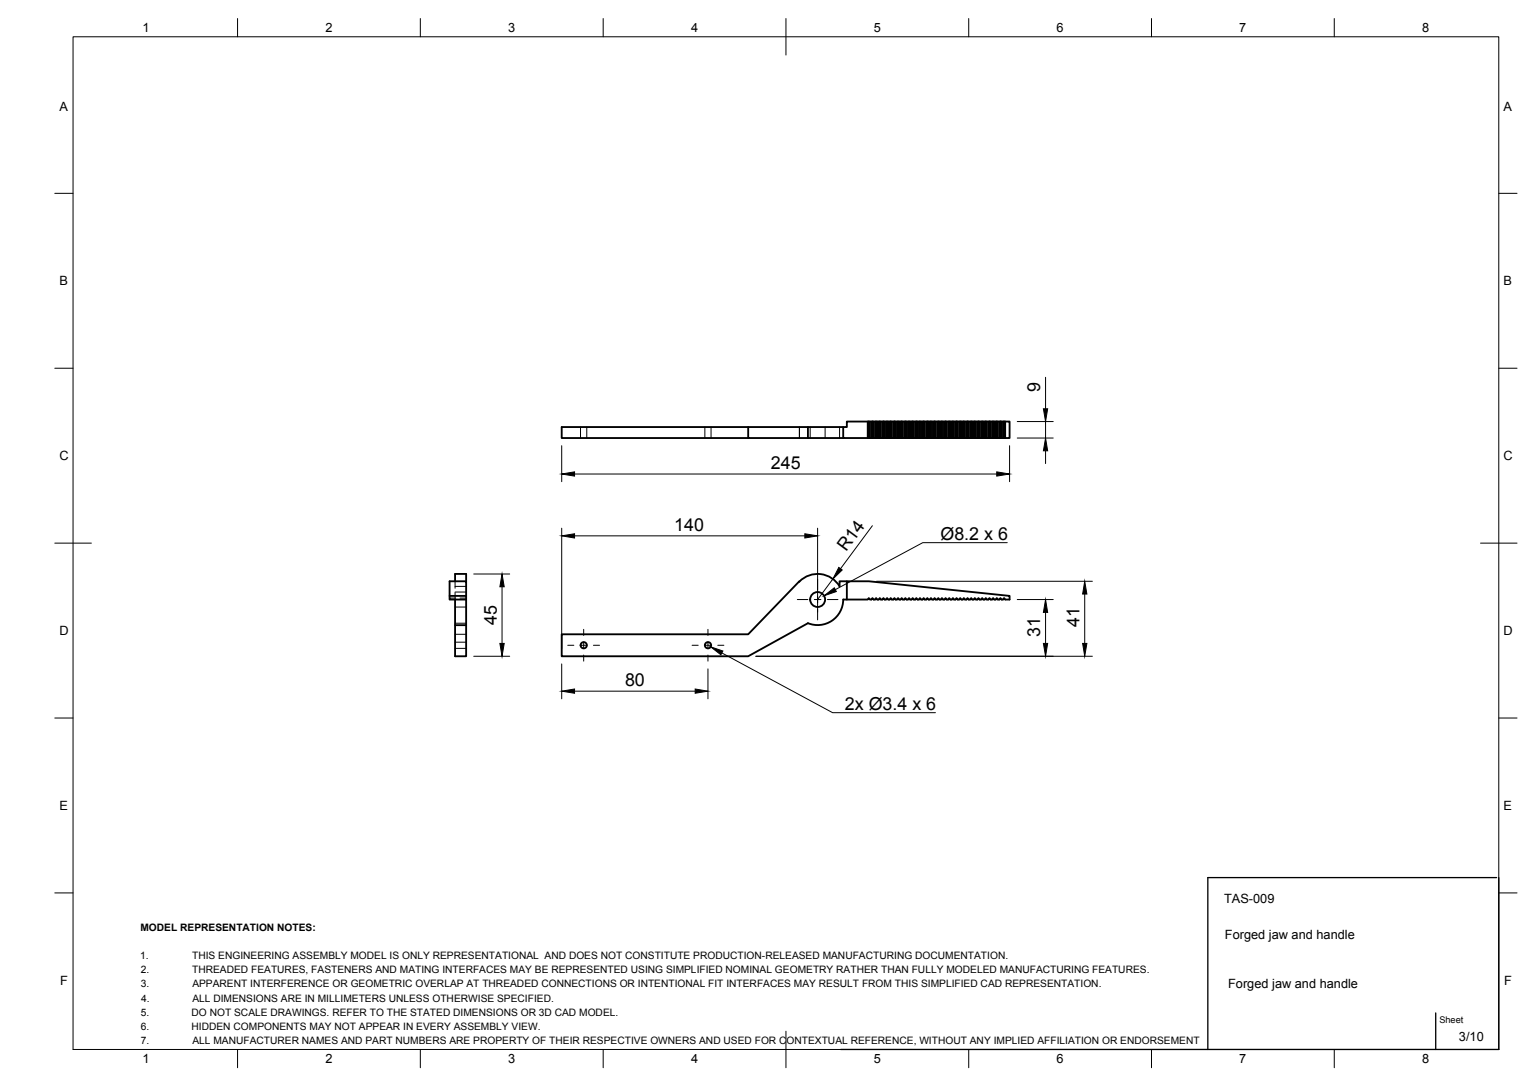
ISO-10303-21;
HEADER;
/* Generated by software containing ST-Developer
 * from STEP Tools, Inc. (www.steptools.com) 
 */

FILE_DESCRIPTION(
/* description */ (''),
/* implementation_level */ '2;1');

FILE_NAME(
/* name */ 'Forged jaw and handle.step',
/* time_stamp */ '2026-11-12T00:53:40-08:00',
/* author */ (''),
/* organization */ (''),
/* preprocessor_version */ 'ST-DEVELOPER v20.2',
/* originating_system */ 'Autodesk Translation Framework v15.17.0.0',
/* authorisation */ '');

FILE_SCHEMA (('AUTOMOTIVE_DESIGN { 1 0 10303 214 3 1 1 }'));
ENDSEC;

DATA;
#10=MECHANICAL_DESIGN_GEOMETRIC_PRESENTATION_REPRESENTATION('',(#572),#22129);
#554=SHAPE_REPRESENTATION_RELATIONSHIP('SRR','None',#22173,#563);
#563=ADVANCED_BREP_SHAPE_REPRESENTATION('',(#581),#22119);
#572=STYLED_ITEM('',(#22232),#581);
#581=MANIFOLD_SOLID_BREP('Body1',#8803);
#590=FACE_BOUND('',#1511,.T.);
#591=FACE_BOUND('',#1512,.T.);
#592=FACE_BOUND('',#1513,.T.);
#593=FACE_BOUND('',#1522,.T.);
#594=FACE_BOUND('',#1523,.T.);
#595=FACE_BOUND('',#1524,.T.);
#651=PLANE('',#8923);
#652=PLANE('',#8924);
#653=PLANE('',#8925);
#654=PLANE('',#8926);
#655=PLANE('',#8927);
#656=PLANE('',#8928);
#657=PLANE('',#8929);
#658=PLANE('',#8930);
#659=PLANE('',#8931);
#660=PLANE('',#8932);
#661=PLANE('',#8933);
#662=PLANE('',#8934);
#663=PLANE('',#8935);
#664=PLANE('',#8936);
#665=PLANE('',#8937);
#666=PLANE('',#8938);
#667=PLANE('',#8939);
#668=PLANE('',#8940);
#669=PLANE('',#8941);
#670=PLANE('',#8942);
#671=PLANE('',#8943);
#672=PLANE('',#8944);
#673=PLANE('',#8945);
#674=PLANE('',#8946);
#675=PLANE('',#8947);
#676=PLANE('',#8948);
#677=PLANE('',#8949);
#678=PLANE('',#8950);
#679=PLANE('',#8951);
#680=PLANE('',#8952);
#681=PLANE('',#8953);
#682=PLANE('',#8954);
#683=PLANE('',#8955);
#684=PLANE('',#8956);
#685=PLANE('',#8957);
#686=PLANE('',#8958);
#687=PLANE('',#8959);
#688=PLANE('',#8960);
#689=PLANE('',#8961);
#690=PLANE('',#8962);
#691=PLANE('',#8963);
#692=PLANE('',#8964);
#693=PLANE('',#8965);
#694=PLANE('',#8966);
#695=PLANE('',#8967);
#696=PLANE('',#8968);
#697=PLANE('',#8969);
#698=PLANE('',#8970);
#699=PLANE('',#8971);
#700=PLANE('',#8972);
#701=PLANE('',#8973);
#702=PLANE('',#8974);
#703=PLANE('',#8975);
#704=PLANE('',#8976);
#705=PLANE('',#8977);
#706=PLANE('',#8978);
#707=PLANE('',#8979);
#708=PLANE('',#8980);
#709=PLANE('',#8981);
#710=PLANE('',#8982);
#711=PLANE('',#8983);
#712=PLANE('',#8984);
#713=PLANE('',#8985);
#714=PLANE('',#8986);
#715=PLANE('',#8987);
#716=PLANE('',#8988);
#717=PLANE('',#8989);
#718=PLANE('',#8990);
#719=PLANE('',#8991);
#720=PLANE('',#8992);
#721=PLANE('',#8993);
#722=PLANE('',#8994);
#723=PLANE('',#8995);
#724=PLANE('',#8996);
#725=PLANE('',#8997);
#726=PLANE('',#8998);
#727=PLANE('',#8999);
#728=PLANE('',#9000);
#729=PLANE('',#9001);
#730=PLANE('',#9002);
#731=PLANE('',#9003);
#732=PLANE('',#9004);
#733=PLANE('',#9005);
#734=PLANE('',#9006);
#735=PLANE('',#9007);
#736=PLANE('',#9008);
#737=PLANE('',#9009);
#738=PLANE('',#9010);
#739=PLANE('',#9011);
#740=PLANE('',#9012);
#741=PLANE('',#9013);
#742=PLANE('',#9014);
#743=PLANE('',#9015);
#744=PLANE('',#9016);
#745=PLANE('',#9017);
#746=PLANE('',#9018);
#747=PLANE('',#9019);
#748=PLANE('',#9020);
#749=PLANE('',#9021);
#750=PLANE('',#9022);
#751=PLANE('',#9023);
#752=PLANE('',#9024);
#753=PLANE('',#9025);
#754=PLANE('',#9026);
#755=PLANE('',#9027);
#756=PLANE('',#9028);
#757=PLANE('',#9029);
#758=PLANE('',#9030);
#759=PLANE('',#9031);
#760=PLANE('',#9032);
#761=PLANE('',#9033);
#762=PLANE('',#9034);
#763=PLANE('',#9035);
#764=PLANE('',#9036);
#765=PLANE('',#9037);
#766=PLANE('',#9038);
#767=PLANE('',#9039);
#768=PLANE('',#9040);
#769=PLANE('',#9041);
#770=PLANE('',#9042);
#771=PLANE('',#9043);
#772=PLANE('',#9044);
#773=PLANE('',#9049);
#774=PLANE('',#9050);
#775=PLANE('',#9051);
#776=PLANE('',#9052);
#777=PLANE('',#9053);
#778=PLANE('',#9054);
#779=PLANE('',#9055);
#903=FACE_OUTER_BOUND('',#1386,.T.);
#904=FACE_OUTER_BOUND('',#1387,.T.);
#905=FACE_OUTER_BOUND('',#1388,.T.);
#906=FACE_OUTER_BOUND('',#1389,.T.);
#907=FACE_OUTER_BOUND('',#1390,.T.);
#908=FACE_OUTER_BOUND('',#1391,.T.);
#909=FACE_OUTER_BOUND('',#1392,.T.);
#910=FACE_OUTER_BOUND('',#1393,.T.);
#911=FACE_OUTER_BOUND('',#1394,.T.);
#912=FACE_OUTER_BOUND('',#1395,.T.);
#913=FACE_OUTER_BOUND('',#1396,.T.);
#914=FACE_OUTER_BOUND('',#1397,.T.);
#915=FACE_OUTER_BOUND('',#1398,.T.);
#916=FACE_OUTER_BOUND('',#1399,.T.);
#917=FACE_OUTER_BOUND('',#1400,.T.);
#918=FACE_OUTER_BOUND('',#1401,.T.);
#919=FACE_OUTER_BOUND('',#1402,.T.);
#920=FACE_OUTER_BOUND('',#1403,.T.);
#921=FACE_OUTER_BOUND('',#1404,.T.);
#922=FACE_OUTER_BOUND('',#1405,.T.);
#923=FACE_OUTER_BOUND('',#1406,.T.);
#924=FACE_OUTER_BOUND('',#1407,.T.);
#925=FACE_OUTER_BOUND('',#1408,.T.);
#926=FACE_OUTER_BOUND('',#1409,.T.);
#927=FACE_OUTER_BOUND('',#1410,.T.);
#928=FACE_OUTER_BOUND('',#1411,.T.);
#929=FACE_OUTER_BOUND('',#1412,.T.);
#930=FACE_OUTER_BOUND('',#1413,.T.);
#931=FACE_OUTER_BOUND('',#1414,.T.);
#932=FACE_OUTER_BOUND('',#1415,.T.);
#933=FACE_OUTER_BOUND('',#1416,.T.);
#934=FACE_OUTER_BOUND('',#1417,.T.);
#935=FACE_OUTER_BOUND('',#1418,.T.);
#936=FACE_OUTER_BOUND('',#1419,.T.);
#937=FACE_OUTER_BOUND('',#1420,.T.);
#938=FACE_OUTER_BOUND('',#1421,.T.);
#939=FACE_OUTER_BOUND('',#1422,.T.);
#940=FACE_OUTER_BOUND('',#1423,.T.);
#941=FACE_OUTER_BOUND('',#1424,.T.);
#942=FACE_OUTER_BOUND('',#1425,.T.);
#943=FACE_OUTER_BOUND('',#1426,.T.);
#944=FACE_OUTER_BOUND('',#1427,.T.);
#945=FACE_OUTER_BOUND('',#1428,.T.);
#946=FACE_OUTER_BOUND('',#1429,.T.);
#947=FACE_OUTER_BOUND('',#1430,.T.);
#948=FACE_OUTER_BOUND('',#1431,.T.);
#949=FACE_OUTER_BOUND('',#1432,.T.);
#950=FACE_OUTER_BOUND('',#1433,.T.);
#951=FACE_OUTER_BOUND('',#1434,.T.);
#952=FACE_OUTER_BOUND('',#1435,.T.);
#953=FACE_OUTER_BOUND('',#1436,.T.);
#954=FACE_OUTER_BOUND('',#1437,.T.);
#955=FACE_OUTER_BOUND('',#1438,.T.);
#956=FACE_OUTER_BOUND('',#1439,.T.);
#957=FACE_OUTER_BOUND('',#1440,.T.);
#958=FACE_OUTER_BOUND('',#1441,.T.);
#959=FACE_OUTER_BOUND('',#1442,.T.);
#960=FACE_OUTER_BOUND('',#1443,.T.);
#961=FACE_OUTER_BOUND('',#1444,.T.);
#962=FACE_OUTER_BOUND('',#1445,.T.);
#963=FACE_OUTER_BOUND('',#1446,.T.);
#964=FACE_OUTER_BOUND('',#1447,.T.);
#965=FACE_OUTER_BOUND('',#1448,.T.);
#966=FACE_OUTER_BOUND('',#1449,.T.);
#967=FACE_OUTER_BOUND('',#1450,.T.);
#968=FACE_OUTER_BOUND('',#1451,.T.);
#969=FACE_OUTER_BOUND('',#1452,.T.);
#970=FACE_OUTER_BOUND('',#1453,.T.);
#971=FACE_OUTER_BOUND('',#1454,.T.);
#972=FACE_OUTER_BOUND('',#1455,.T.);
#973=FACE_OUTER_BOUND('',#1456,.T.);
#974=FACE_OUTER_BOUND('',#1457,.T.);
#975=FACE_OUTER_BOUND('',#1458,.T.);
#976=FACE_OUTER_BOUND('',#1459,.T.);
#977=FACE_OUTER_BOUND('',#1460,.T.);
#978=FACE_OUTER_BOUND('',#1461,.T.);
#979=FACE_OUTER_BOUND('',#1462,.T.);
#980=FACE_OUTER_BOUND('',#1463,.T.);
#981=FACE_OUTER_BOUND('',#1464,.T.);
#982=FACE_OUTER_BOUND('',#1465,.T.);
#983=FACE_OUTER_BOUND('',#1466,.T.);
#984=FACE_OUTER_BOUND('',#1467,.T.);
#985=FACE_OUTER_BOUND('',#1468,.T.);
#986=FACE_OUTER_BOUND('',#1469,.T.);
#987=FACE_OUTER_BOUND('',#1470,.T.);
#988=FACE_OUTER_BOUND('',#1471,.T.);
#989=FACE_OUTER_BOUND('',#1472,.T.);
#990=FACE_OUTER_BOUND('',#1473,.T.);
#991=FACE_OUTER_BOUND('',#1474,.T.);
#992=FACE_OUTER_BOUND('',#1475,.T.);
#993=FACE_OUTER_BOUND('',#1476,.T.);
#994=FACE_OUTER_BOUND('',#1477,.T.);
#995=FACE_OUTER_BOUND('',#1478,.T.);
#996=FACE_OUTER_BOUND('',#1479,.T.);
#997=FACE_OUTER_BOUND('',#1480,.T.);
#998=FACE_OUTER_BOUND('',#1481,.T.);
#999=FACE_OUTER_BOUND('',#1482,.T.);
#1000=FACE_OUTER_BOUND('',#1483,.T.);
#1001=FACE_OUTER_BOUND('',#1484,.T.);
#1002=FACE_OUTER_BOUND('',#1485,.T.);
#1003=FACE_OUTER_BOUND('',#1486,.T.);
#1004=FACE_OUTER_BOUND('',#1487,.T.);
#1005=FACE_OUTER_BOUND('',#1488,.T.);
#1006=FACE_OUTER_BOUND('',#1489,.T.);
#1007=FACE_OUTER_BOUND('',#1490,.T.);
#1008=FACE_OUTER_BOUND('',#1491,.T.);
#1009=FACE_OUTER_BOUND('',#1492,.T.);
#1010=FACE_OUTER_BOUND('',#1493,.T.);
#1011=FACE_OUTER_BOUND('',#1494,.T.);
#1012=FACE_OUTER_BOUND('',#1495,.T.);
#1013=FACE_OUTER_BOUND('',#1496,.T.);
#1014=FACE_OUTER_BOUND('',#1497,.T.);
#1015=FACE_OUTER_BOUND('',#1498,.T.);
#1016=FACE_OUTER_BOUND('',#1499,.T.);
#1017=FACE_OUTER_BOUND('',#1500,.T.);
#1018=FACE_OUTER_BOUND('',#1501,.T.);
#1019=FACE_OUTER_BOUND('',#1502,.T.);
#1020=FACE_OUTER_BOUND('',#1503,.T.);
#1021=FACE_OUTER_BOUND('',#1504,.T.);
#1022=FACE_OUTER_BOUND('',#1505,.T.);
#1023=FACE_OUTER_BOUND('',#1506,.T.);
#1024=FACE_OUTER_BOUND('',#1507,.T.);
#1025=FACE_OUTER_BOUND('',#1508,.T.);
#1026=FACE_OUTER_BOUND('',#1509,.T.);
#1027=FACE_OUTER_BOUND('',#1510,.T.);
#1028=FACE_OUTER_BOUND('',#1514,.T.);
#1029=FACE_OUTER_BOUND('',#1515,.T.);
#1030=FACE_OUTER_BOUND('',#1516,.T.);
#1031=FACE_OUTER_BOUND('',#1517,.T.);
#1032=FACE_OUTER_BOUND('',#1518,.T.);
#1033=FACE_OUTER_BOUND('',#1519,.T.);
#1034=FACE_OUTER_BOUND('',#1520,.T.);
#1035=FACE_OUTER_BOUND('',#1521,.T.);
#1036=FACE_OUTER_BOUND('',#1525,.T.);
#1386=EDGE_LOOP('',(#5646,#5647,#5648,#5649));
#1387=EDGE_LOOP('',(#5650,#5651,#5652,#5653));
#1388=EDGE_LOOP('',(#5654,#5655,#5656,#5657));
#1389=EDGE_LOOP('',(#5658,#5659,#5660,#5661));
#1390=EDGE_LOOP('',(#5662,#5663,#5664,#5665));
#1391=EDGE_LOOP('',(#5666,#5667,#5668,#5669));
#1392=EDGE_LOOP('',(#5670,#5671,#5672,#5673));
#1393=EDGE_LOOP('',(#5674,#5675,#5676,#5677));
#1394=EDGE_LOOP('',(#5678,#5679,#5680,#5681));
#1395=EDGE_LOOP('',(#5682,#5683,#5684,#5685));
#1396=EDGE_LOOP('',(#5686,#5687,#5688,#5689));
#1397=EDGE_LOOP('',(#5690,#5691,#5692,#5693));
#1398=EDGE_LOOP('',(#5694,#5695,#5696,#5697));
#1399=EDGE_LOOP('',(#5698,#5699,#5700,#5701));
#1400=EDGE_LOOP('',(#5702,#5703,#5704,#5705));
#1401=EDGE_LOOP('',(#5706,#5707,#5708,#5709));
#1402=EDGE_LOOP('',(#5710,#5711,#5712,#5713));
#1403=EDGE_LOOP('',(#5714,#5715,#5716,#5717));
#1404=EDGE_LOOP('',(#5718,#5719,#5720,#5721));
#1405=EDGE_LOOP('',(#5722,#5723,#5724,#5725));
#1406=EDGE_LOOP('',(#5726,#5727,#5728,#5729));
#1407=EDGE_LOOP('',(#5730,#5731,#5732,#5733));
#1408=EDGE_LOOP('',(#5734,#5735,#5736,#5737));
#1409=EDGE_LOOP('',(#5738,#5739,#5740,#5741));
#1410=EDGE_LOOP('',(#5742,#5743,#5744,#5745));
#1411=EDGE_LOOP('',(#5746,#5747,#5748,#5749));
#1412=EDGE_LOOP('',(#5750,#5751,#5752,#5753));
#1413=EDGE_LOOP('',(#5754,#5755,#5756,#5757));
#1414=EDGE_LOOP('',(#5758,#5759,#5760,#5761));
#1415=EDGE_LOOP('',(#5762,#5763,#5764,#5765));
#1416=EDGE_LOOP('',(#5766,#5767,#5768,#5769));
#1417=EDGE_LOOP('',(#5770,#5771,#5772,#5773));
#1418=EDGE_LOOP('',(#5774,#5775,#5776,#5777));
#1419=EDGE_LOOP('',(#5778,#5779,#5780,#5781));
#1420=EDGE_LOOP('',(#5782,#5783,#5784,#5785));
#1421=EDGE_LOOP('',(#5786,#5787,#5788,#5789));
#1422=EDGE_LOOP('',(#5790,#5791,#5792,#5793));
#1423=EDGE_LOOP('',(#5794,#5795,#5796,#5797));
#1424=EDGE_LOOP('',(#5798,#5799,#5800,#5801));
#1425=EDGE_LOOP('',(#5802,#5803,#5804,#5805));
#1426=EDGE_LOOP('',(#5806,#5807,#5808,#5809));
#1427=EDGE_LOOP('',(#5810,#5811,#5812,#5813));
#1428=EDGE_LOOP('',(#5814,#5815,#5816,#5817));
#1429=EDGE_LOOP('',(#5818,#5819,#5820,#5821));
#1430=EDGE_LOOP('',(#5822,#5823,#5824,#5825));
#1431=EDGE_LOOP('',(#5826,#5827,#5828,#5829));
#1432=EDGE_LOOP('',(#5830,#5831,#5832,#5833));
#1433=EDGE_LOOP('',(#5834,#5835,#5836,#5837));
#1434=EDGE_LOOP('',(#5838,#5839,#5840,#5841));
#1435=EDGE_LOOP('',(#5842,#5843,#5844,#5845));
#1436=EDGE_LOOP('',(#5846,#5847,#5848,#5849));
#1437=EDGE_LOOP('',(#5850,#5851,#5852,#5853));
#1438=EDGE_LOOP('',(#5854,#5855,#5856,#5857));
#1439=EDGE_LOOP('',(#5858,#5859,#5860,#5861));
#1440=EDGE_LOOP('',(#5862,#5863,#5864,#5865));
#1441=EDGE_LOOP('',(#5866,#5867,#5868,#5869));
#1442=EDGE_LOOP('',(#5870,#5871,#5872,#5873));
#1443=EDGE_LOOP('',(#5874,#5875,#5876,#5877));
#1444=EDGE_LOOP('',(#5878,#5879,#5880,#5881));
#1445=EDGE_LOOP('',(#5882,#5883,#5884,#5885));
#1446=EDGE_LOOP('',(#5886,#5887,#5888,#5889));
#1447=EDGE_LOOP('',(#5890,#5891,#5892,#5893));
#1448=EDGE_LOOP('',(#5894,#5895,#5896,#5897));
#1449=EDGE_LOOP('',(#5898,#5899,#5900,#5901));
#1450=EDGE_LOOP('',(#5902,#5903,#5904,#5905));
#1451=EDGE_LOOP('',(#5906,#5907,#5908,#5909));
#1452=EDGE_LOOP('',(#5910,#5911,#5912,#5913));
#1453=EDGE_LOOP('',(#5914,#5915,#5916,#5917));
#1454=EDGE_LOOP('',(#5918,#5919,#5920,#5921));
#1455=EDGE_LOOP('',(#5922,#5923,#5924,#5925));
#1456=EDGE_LOOP('',(#5926,#5927,#5928,#5929));
#1457=EDGE_LOOP('',(#5930,#5931,#5932,#5933));
#1458=EDGE_LOOP('',(#5934,#5935,#5936,#5937));
#1459=EDGE_LOOP('',(#5938,#5939,#5940,#5941));
#1460=EDGE_LOOP('',(#5942,#5943,#5944,#5945));
#1461=EDGE_LOOP('',(#5946,#5947,#5948,#5949));
#1462=EDGE_LOOP('',(#5950,#5951,#5952,#5953));
#1463=EDGE_LOOP('',(#5954,#5955,#5956,#5957));
#1464=EDGE_LOOP('',(#5958,#5959,#5960,#5961));
#1465=EDGE_LOOP('',(#5962,#5963,#5964,#5965,#5966,#5967));
#1466=EDGE_LOOP('',(#5968,#5969,#5970,#5971));
#1467=EDGE_LOOP('',(#5972,#5973,#5974,#5975));
#1468=EDGE_LOOP('',(#5976,#5977,#5978,#5979));
#1469=EDGE_LOOP('',(#5980,#5981,#5982,#5983));
#1470=EDGE_LOOP('',(#5984,#5985,#5986,#5987));
#1471=EDGE_LOOP('',(#5988,#5989,#5990,#5991));
#1472=EDGE_LOOP('',(#5992,#5993,#5994,#5995));
#1473=EDGE_LOOP('',(#5996,#5997,#5998,#5999));
#1474=EDGE_LOOP('',(#6000,#6001,#6002,#6003));
#1475=EDGE_LOOP('',(#6004,#6005,#6006,#6007));
#1476=EDGE_LOOP('',(#6008,#6009,#6010,#6011));
#1477=EDGE_LOOP('',(#6012,#6013,#6014,#6015));
#1478=EDGE_LOOP('',(#6016,#6017,#6018,#6019));
#1479=EDGE_LOOP('',(#6020,#6021,#6022,#6023));
#1480=EDGE_LOOP('',(#6024,#6025,#6026,#6027));
#1481=EDGE_LOOP('',(#6028,#6029,#6030,#6031));
#1482=EDGE_LOOP('',(#6032,#6033,#6034,#6035));
#1483=EDGE_LOOP('',(#6036,#6037,#6038,#6039));
#1484=EDGE_LOOP('',(#6040,#6041,#6042,#6043));
#1485=EDGE_LOOP('',(#6044,#6045,#6046,#6047));
#1486=EDGE_LOOP('',(#6048,#6049,#6050,#6051));
#1487=EDGE_LOOP('',(#6052,#6053,#6054,#6055));
#1488=EDGE_LOOP('',(#6056,#6057,#6058,#6059));
#1489=EDGE_LOOP('',(#6060,#6061,#6062,#6063));
#1490=EDGE_LOOP('',(#6064,#6065,#6066,#6067));
#1491=EDGE_LOOP('',(#6068,#6069,#6070,#6071));
#1492=EDGE_LOOP('',(#6072,#6073,#6074,#6075));
#1493=EDGE_LOOP('',(#6076,#6077,#6078,#6079));
#1494=EDGE_LOOP('',(#6080,#6081,#6082,#6083));
#1495=EDGE_LOOP('',(#6084,#6085,#6086,#6087));
#1496=EDGE_LOOP('',(#6088,#6089,#6090,#6091));
#1497=EDGE_LOOP('',(#6092,#6093,#6094,#6095));
#1498=EDGE_LOOP('',(#6096,#6097,#6098,#6099));
#1499=EDGE_LOOP('',(#6100,#6101,#6102,#6103));
#1500=EDGE_LOOP('',(#6104,#6105,#6106,#6107));
#1501=EDGE_LOOP('',(#6108,#6109,#6110,#6111));
#1502=EDGE_LOOP('',(#6112,#6113,#6114,#6115));
#1503=EDGE_LOOP('',(#6116,#6117,#6118,#6119));
#1504=EDGE_LOOP('',(#6120,#6121,#6122,#6123,#6124,#6125,#6126,#6127,#6128,
#6129,#6130,#6131,#6132,#6133,#6134,#6135,#6136,#6137,#6138,#6139,#6140,
#6141,#6142,#6143,#6144,#6145,#6146,#6147,#6148,#6149,#6150,#6151,#6152,
#6153,#6154,#6155,#6156,#6157,#6158,#6159,#6160,#6161,#6162,#6163,#6164,
#6165,#6166,#6167,#6168,#6169,#6170,#6171,#6172,#6173,#6174,#6175,#6176,
#6177,#6178,#6179,#6180,#6181,#6182,#6183,#6184,#6185,#6186,#6187,#6188,
#6189,#6190,#6191,#6192,#6193,#6194,#6195,#6196,#6197,#6198,#6199,#6200,
#6201,#6202,#6203,#6204,#6205,#6206,#6207,#6208,#6209,#6210,#6211,#6212,
#6213,#6214,#6215,#6216,#6217,#6218,#6219,#6220,#6221,#6222,#6223,#6224,
#6225,#6226,#6227,#6228,#6229,#6230,#6231,#6232,#6233,#6234,#6235,#6236,
#6237,#6238));
#1505=EDGE_LOOP('',(#6239,#6240,#6241,#6242));
#1506=EDGE_LOOP('',(#6243,#6244,#6245,#6246));
#1507=EDGE_LOOP('',(#6247,#6248,#6249,#6250));
#1508=EDGE_LOOP('',(#6251,#6252,#6253,#6254));
#1509=EDGE_LOOP('',(#6255,#6256,#6257,#6258,#6259,#6260));
#1510=EDGE_LOOP('',(#6261,#6262,#6263,#6264,#6265,#6266,#6267,#6268,#6269,
#6270,#6271,#6272));
#1511=EDGE_LOOP('',(#6273));
#1512=EDGE_LOOP('',(#6274));
#1513=EDGE_LOOP('',(#6275));
#1514=EDGE_LOOP('',(#6276,#6277,#6278,#6279));
#1515=EDGE_LOOP('',(#6280,#6281,#6282,#6283));
#1516=EDGE_LOOP('',(#6284,#6285,#6286,#6287));
#1517=EDGE_LOOP('',(#6288,#6289,#6290,#6291));
#1518=EDGE_LOOP('',(#6292,#6293,#6294,#6295));
#1519=EDGE_LOOP('',(#6296,#6297,#6298,#6299));
#1520=EDGE_LOOP('',(#6300,#6301,#6302,#6303));
#1521=EDGE_LOOP('',(#6304,#6305,#6306,#6307,#6308,#6309,#6310,#6311,#6312,
#6313,#6314,#6315,#6316,#6317,#6318,#6319,#6320,#6321,#6322,#6323,#6324,
#6325,#6326,#6327,#6328,#6329,#6330,#6331,#6332,#6333,#6334,#6335,#6336,
#6337,#6338,#6339,#6340,#6341,#6342,#6343,#6344,#6345,#6346,#6347,#6348,
#6349,#6350,#6351,#6352,#6353,#6354,#6355,#6356,#6357,#6358,#6359,#6360,
#6361,#6362,#6363,#6364,#6365,#6366,#6367,#6368,#6369,#6370,#6371,#6372,
#6373,#6374,#6375,#6376,#6377,#6378,#6379,#6380,#6381,#6382,#6383,#6384,
#6385,#6386,#6387,#6388,#6389,#6390,#6391,#6392,#6393,#6394,#6395,#6396,
#6397,#6398,#6399,#6400,#6401,#6402,#6403,#6404,#6405,#6406,#6407,#6408,
#6409,#6410,#6411,#6412,#6413,#6414,#6415,#6416,#6417,#6418,#6419,#6420,
#6421,#6422,#6423,#6424,#6425,#6426,#6427,#6428,#6429,#6430));
#1522=EDGE_LOOP('',(#6431));
#1523=EDGE_LOOP('',(#6432));
#1524=EDGE_LOOP('',(#6433));
#1525=EDGE_LOOP('',(#6434,#6435,#6436,#6437));
#1930=LINE('',#11412,#2660);
#1931=LINE('',#11418,#2661);
#1932=LINE('',#11424,#2662);
#1933=LINE('',#11429,#2663);
#1934=LINE('',#11431,#2664);
#1935=LINE('',#11433,#2665);
#1936=LINE('',#11434,#2666);
#1937=LINE('',#11438,#2667);
#1938=LINE('',#11439,#2668);
#1939=LINE('',#11440,#2669);
#1940=LINE('',#11444,#2670);
#1941=LINE('',#11446,#2671);
#1942=LINE('',#11448,#2672);
#1943=LINE('',#11449,#2673);
#1944=LINE('',#11453,#2674);
#1945=LINE('',#11454,#2675);
#1946=LINE('',#11455,#2676);
#1947=LINE('',#11459,#2677);
#1948=LINE('',#11461,#2678);
#1949=LINE('',#11463,#2679);
#1950=LINE('',#11464,#2680);
#1951=LINE('',#11468,#2681);
#1952=LINE('',#11469,#2682);
#1953=LINE('',#11470,#2683);
#1954=LINE('',#11474,#2684);
#1955=LINE('',#11476,#2685);
#1956=LINE('',#11478,#2686);
#1957=LINE('',#11479,#2687);
#1958=LINE('',#11483,#2688);
#1959=LINE('',#11484,#2689);
#1960=LINE('',#11485,#2690);
#1961=LINE('',#11489,#2691);
#1962=LINE('',#11491,#2692);
#1963=LINE('',#11493,#2693);
#1964=LINE('',#11494,#2694);
#1965=LINE('',#11498,#2695);
#1966=LINE('',#11499,#2696);
#1967=LINE('',#11500,#2697);
#1968=LINE('',#11504,#2698);
#1969=LINE('',#11506,#2699);
#1970=LINE('',#11508,#2700);
#1971=LINE('',#11509,#2701);
#1972=LINE('',#11513,#2702);
#1973=LINE('',#11514,#2703);
#1974=LINE('',#11515,#2704);
#1975=LINE('',#11519,#2705);
#1976=LINE('',#11521,#2706);
#1977=LINE('',#11523,#2707);
#1978=LINE('',#11524,#2708);
#1979=LINE('',#11528,#2709);
#1980=LINE('',#11529,#2710);
#1981=LINE('',#11530,#2711);
#1982=LINE('',#11534,#2712);
#1983=LINE('',#11536,#2713);
#1984=LINE('',#11538,#2714);
#1985=LINE('',#11539,#2715);
#1986=LINE('',#11543,#2716);
#1987=LINE('',#11544,#2717);
#1988=LINE('',#11545,#2718);
#1989=LINE('',#11549,#2719);
#1990=LINE('',#11551,#2720);
#1991=LINE('',#11553,#2721);
#1992=LINE('',#11554,#2722);
#1993=LINE('',#11558,#2723);
#1994=LINE('',#11559,#2724);
#1995=LINE('',#11560,#2725);
#1996=LINE('',#11564,#2726);
#1997=LINE('',#11566,#2727);
#1998=LINE('',#11568,#2728);
#1999=LINE('',#11569,#2729);
#2000=LINE('',#11573,#2730);
#2001=LINE('',#11574,#2731);
#2002=LINE('',#11575,#2732);
#2003=LINE('',#11579,#2733);
#2004=LINE('',#11581,#2734);
#2005=LINE('',#11583,#2735);
#2006=LINE('',#11584,#2736);
#2007=LINE('',#11588,#2737);
#2008=LINE('',#11589,#2738);
#2009=LINE('',#11590,#2739);
#2010=LINE('',#11594,#2740);
#2011=LINE('',#11596,#2741);
#2012=LINE('',#11598,#2742);
#2013=LINE('',#11599,#2743);
#2014=LINE('',#11603,#2744);
#2015=LINE('',#11604,#2745);
#2016=LINE('',#11605,#2746);
#2017=LINE('',#11609,#2747);
#2018=LINE('',#11611,#2748);
#2019=LINE('',#11613,#2749);
#2020=LINE('',#11614,#2750);
#2021=LINE('',#11618,#2751);
#2022=LINE('',#11619,#2752);
#2023=LINE('',#11620,#2753);
#2024=LINE('',#11624,#2754);
#2025=LINE('',#11626,#2755);
#2026=LINE('',#11628,#2756);
#2027=LINE('',#11629,#2757);
#2028=LINE('',#11633,#2758);
#2029=LINE('',#11634,#2759);
#2030=LINE('',#11635,#2760);
#2031=LINE('',#11639,#2761);
#2032=LINE('',#11641,#2762);
#2033=LINE('',#11643,#2763);
#2034=LINE('',#11644,#2764);
#2035=LINE('',#11648,#2765);
#2036=LINE('',#11649,#2766);
#2037=LINE('',#11650,#2767);
#2038=LINE('',#11654,#2768);
#2039=LINE('',#11656,#2769);
#2040=LINE('',#11658,#2770);
#2041=LINE('',#11659,#2771);
#2042=LINE('',#11663,#2772);
#2043=LINE('',#11664,#2773);
#2044=LINE('',#11665,#2774);
#2045=LINE('',#11669,#2775);
#2046=LINE('',#11671,#2776);
#2047=LINE('',#11673,#2777);
#2048=LINE('',#11674,#2778);
#2049=LINE('',#11678,#2779);
#2050=LINE('',#11679,#2780);
#2051=LINE('',#11680,#2781);
#2052=LINE('',#11684,#2782);
#2053=LINE('',#11686,#2783);
#2054=LINE('',#11688,#2784);
#2055=LINE('',#11689,#2785);
#2056=LINE('',#11693,#2786);
#2057=LINE('',#11694,#2787);
#2058=LINE('',#11695,#2788);
#2059=LINE('',#11699,#2789);
#2060=LINE('',#11701,#2790);
#2061=LINE('',#11703,#2791);
#2062=LINE('',#11704,#2792);
#2063=LINE('',#11708,#2793);
#2064=LINE('',#11709,#2794);
#2065=LINE('',#11710,#2795);
#2066=LINE('',#11714,#2796);
#2067=LINE('',#11716,#2797);
#2068=LINE('',#11718,#2798);
#2069=LINE('',#11719,#2799);
#2070=LINE('',#11723,#2800);
#2071=LINE('',#11724,#2801);
#2072=LINE('',#11725,#2802);
#2073=LINE('',#11729,#2803);
#2074=LINE('',#11731,#2804);
#2075=LINE('',#11733,#2805);
#2076=LINE('',#11734,#2806);
#2077=LINE('',#11738,#2807);
#2078=LINE('',#11739,#2808);
#2079=LINE('',#11740,#2809);
#2080=LINE('',#11744,#2810);
#2081=LINE('',#11746,#2811);
#2082=LINE('',#11748,#2812);
#2083=LINE('',#11749,#2813);
#2084=LINE('',#11753,#2814);
#2085=LINE('',#11754,#2815);
#2086=LINE('',#11755,#2816);
#2087=LINE('',#11759,#2817);
#2088=LINE('',#11761,#2818);
#2089=LINE('',#11763,#2819);
#2090=LINE('',#11764,#2820);
#2091=LINE('',#11768,#2821);
#2092=LINE('',#11769,#2822);
#2093=LINE('',#11770,#2823);
#2094=LINE('',#11774,#2824);
#2095=LINE('',#11776,#2825);
#2096=LINE('',#11778,#2826);
#2097=LINE('',#11779,#2827);
#2098=LINE('',#11783,#2828);
#2099=LINE('',#11784,#2829);
#2100=LINE('',#11785,#2830);
#2101=LINE('',#11789,#2831);
#2102=LINE('',#11791,#2832);
#2103=LINE('',#11793,#2833);
#2104=LINE('',#11794,#2834);
#2105=LINE('',#11798,#2835);
#2106=LINE('',#11799,#2836);
#2107=LINE('',#11800,#2837);
#2108=LINE('',#11804,#2838);
#2109=LINE('',#11806,#2839);
#2110=LINE('',#11808,#2840);
#2111=LINE('',#11809,#2841);
#2112=LINE('',#11813,#2842);
#2113=LINE('',#11814,#2843);
#2114=LINE('',#11815,#2844);
#2115=LINE('',#11819,#2845);
#2116=LINE('',#11821,#2846);
#2117=LINE('',#11823,#2847);
#2118=LINE('',#11824,#2848);
#2119=LINE('',#11828,#2849);
#2120=LINE('',#11829,#2850);
#2121=LINE('',#11830,#2851);
#2122=LINE('',#11834,#2852);
#2123=LINE('',#11836,#2853);
#2124=LINE('',#11838,#2854);
#2125=LINE('',#11839,#2855);
#2126=LINE('',#11843,#2856);
#2127=LINE('',#11844,#2857);
#2128=LINE('',#11845,#2858);
#2129=LINE('',#11849,#2859);
#2130=LINE('',#11851,#2860);
#2131=LINE('',#11853,#2861);
#2132=LINE('',#11854,#2862);
#2133=LINE('',#11858,#2863);
#2134=LINE('',#11859,#2864);
#2135=LINE('',#11860,#2865);
#2136=LINE('',#11864,#2866);
#2137=LINE('',#11866,#2867);
#2138=LINE('',#11868,#2868);
#2139=LINE('',#11869,#2869);
#2140=LINE('',#11873,#2870);
#2141=LINE('',#11874,#2871);
#2142=LINE('',#11875,#2872);
#2143=LINE('',#11879,#2873);
#2144=LINE('',#11881,#2874);
#2145=LINE('',#11883,#2875);
#2146=LINE('',#11884,#2876);
#2147=LINE('',#11888,#2877);
#2148=LINE('',#11889,#2878);
#2149=LINE('',#11890,#2879);
#2150=LINE('',#11894,#2880);
#2151=LINE('',#11896,#2881);
#2152=LINE('',#11898,#2882);
#2153=LINE('',#11899,#2883);
#2154=LINE('',#11903,#2884);
#2155=LINE('',#11904,#2885);
#2156=LINE('',#11905,#2886);
#2157=LINE('',#11909,#2887);
#2158=LINE('',#11911,#2888);
#2159=LINE('',#11913,#2889);
#2160=LINE('',#11914,#2890);
#2161=LINE('',#11918,#2891);
#2162=LINE('',#11919,#2892);
#2163=LINE('',#11920,#2893);
#2164=LINE('',#11924,#2894);
#2165=LINE('',#11926,#2895);
#2166=LINE('',#11928,#2896);
#2167=LINE('',#11929,#2897);
#2168=LINE('',#11933,#2898);
#2169=LINE('',#11934,#2899);
#2170=LINE('',#11935,#2900);
#2171=LINE('',#11939,#2901);
#2172=LINE('',#11941,#2902);
#2173=LINE('',#11943,#2903);
#2174=LINE('',#11944,#2904);
#2175=LINE('',#11948,#2905);
#2176=LINE('',#11949,#2906);
#2177=LINE('',#11950,#2907);
#2178=LINE('',#11954,#2908);
#2179=LINE('',#11956,#2909);
#2180=LINE('',#11958,#2910);
#2181=LINE('',#11959,#2911);
#2182=LINE('',#11963,#2912);
#2183=LINE('',#11964,#2913);
#2184=LINE('',#11965,#2914);
#2185=LINE('',#11969,#2915);
#2186=LINE('',#11971,#2916);
#2187=LINE('',#11973,#2917);
#2188=LINE('',#11974,#2918);
#2189=LINE('',#11978,#2919);
#2190=LINE('',#11979,#2920);
#2191=LINE('',#11980,#2921);
#2192=LINE('',#11984,#2922);
#2193=LINE('',#11986,#2923);
#2194=LINE('',#11988,#2924);
#2195=LINE('',#11989,#2925);
#2196=LINE('',#11993,#2926);
#2197=LINE('',#11994,#2927);
#2198=LINE('',#11995,#2928);
#2199=LINE('',#11998,#2929);
#2200=LINE('',#12000,#2930);
#2201=LINE('',#12002,#2931);
#2202=LINE('',#12004,#2932);
#2203=LINE('',#12005,#2933);
#2204=LINE('',#12007,#2934);
#2205=LINE('',#12008,#2935);
#2206=LINE('',#12010,#2936);
#2207=LINE('',#12011,#2937);
#2208=LINE('',#12013,#2938);
#2209=LINE('',#12014,#2939);
#2210=LINE('',#12016,#2940);
#2211=LINE('',#12017,#2941);
#2212=LINE('',#12019,#2942);
#2213=LINE('',#12020,#2943);
#2214=LINE('',#12022,#2944);
#2215=LINE('',#12023,#2945);
#2216=LINE('',#12025,#2946);
#2217=LINE('',#12026,#2947);
#2218=LINE('',#12028,#2948);
#2219=LINE('',#12029,#2949);
#2220=LINE('',#12031,#2950);
#2221=LINE('',#12032,#2951);
#2222=LINE('',#12034,#2952);
#2223=LINE('',#12035,#2953);
#2224=LINE('',#12037,#2954);
#2225=LINE('',#12038,#2955);
#2226=LINE('',#12040,#2956);
#2227=LINE('',#12041,#2957);
#2228=LINE('',#12043,#2958);
#2229=LINE('',#12044,#2959);
#2230=LINE('',#12046,#2960);
#2231=LINE('',#12047,#2961);
#2232=LINE('',#12049,#2962);
#2233=LINE('',#12050,#2963);
#2234=LINE('',#12052,#2964);
#2235=LINE('',#12053,#2965);
#2236=LINE('',#12055,#2966);
#2237=LINE('',#12056,#2967);
#2238=LINE('',#12058,#2968);
#2239=LINE('',#12059,#2969);
#2240=LINE('',#12061,#2970);
#2241=LINE('',#12062,#2971);
#2242=LINE('',#12064,#2972);
#2243=LINE('',#12065,#2973);
#2244=LINE('',#12067,#2974);
#2245=LINE('',#12068,#2975);
#2246=LINE('',#12070,#2976);
#2247=LINE('',#12071,#2977);
#2248=LINE('',#12073,#2978);
#2249=LINE('',#12074,#2979);
#2250=LINE('',#12076,#2980);
#2251=LINE('',#12077,#2981);
#2252=LINE('',#12079,#2982);
#2253=LINE('',#12080,#2983);
#2254=LINE('',#12082,#2984);
#2255=LINE('',#12083,#2985);
#2256=LINE('',#12085,#2986);
#2257=LINE('',#12086,#2987);
#2258=LINE('',#12088,#2988);
#2259=LINE('',#12089,#2989);
#2260=LINE('',#12092,#2990);
#2261=LINE('',#12094,#2991);
#2262=LINE('',#12095,#2992);
#2263=LINE('',#12097,#2993);
#2264=LINE('',#12098,#2994);
#2265=LINE('',#12100,#2995);
#2266=LINE('',#12101,#2996);
#2267=LINE('',#12103,#2997);
#2268=LINE('',#12104,#2998);
#2269=LINE('',#12106,#2999);
#2270=LINE('',#12107,#3000);
#2271=LINE('',#12109,#3001);
#2272=LINE('',#12110,#3002);
#2273=LINE('',#12112,#3003);
#2274=LINE('',#12113,#3004);
#2275=LINE('',#12115,#3005);
#2276=LINE('',#12116,#3006);
#2277=LINE('',#12118,#3007);
#2278=LINE('',#12119,#3008);
#2279=LINE('',#12121,#3009);
#2280=LINE('',#12122,#3010);
#2281=LINE('',#12125,#3011);
#2282=LINE('',#12127,#3012);
#2283=LINE('',#12129,#3013);
#2284=LINE('',#12130,#3014);
#2285=LINE('',#12133,#3015);
#2286=LINE('',#12134,#3016);
#2287=LINE('',#12138,#3017);
#2288=LINE('',#12140,#3018);
#2289=LINE('',#12142,#3019);
#2290=LINE('',#12143,#3020);
#2291=LINE('',#12146,#3021);
#2292=LINE('',#12147,#3022);
#2293=LINE('',#12150,#3023);
#2294=LINE('',#12151,#3024);
#2295=LINE('',#12153,#3025);
#2296=LINE('',#12154,#3026);
#2297=LINE('',#12159,#3027);
#2298=LINE('',#12161,#3028);
#2299=LINE('',#12163,#3029);
#2300=LINE('',#12165,#3030);
#2301=LINE('',#12167,#3031);
#2302=LINE('',#12169,#3032);
#2303=LINE('',#12174,#3033);
#2304=LINE('',#12177,#3034);
#2305=LINE('',#12179,#3035);
#2306=LINE('',#12180,#3036);
#2307=LINE('',#12183,#3037);
#2308=LINE('',#12184,#3038);
#2309=LINE('',#12187,#3039);
#2310=LINE('',#12188,#3040);
#2311=LINE('',#12191,#3041);
#2312=LINE('',#12192,#3042);
#2313=LINE('',#12195,#3043);
#2314=LINE('',#12196,#3044);
#2315=LINE('',#12198,#3045);
#2660=VECTOR('',#9508,0.17);
#2661=VECTOR('',#9515,0.17);
#2662=VECTOR('',#9522,0.41);
#2663=VECTOR('',#9527,1.);
#2664=VECTOR('',#9528,1.);
#2665=VECTOR('',#9529,1.);
#2666=VECTOR('',#9530,1.);
#2667=VECTOR('',#9533,1.);
#2668=VECTOR('',#9534,1.);
#2669=VECTOR('',#9535,1.);
#2670=VECTOR('',#9538,1.);
#2671=VECTOR('',#9539,1.);
#2672=VECTOR('',#9540,1.);
#2673=VECTOR('',#9541,1.);
#2674=VECTOR('',#9544,1.);
#2675=VECTOR('',#9545,1.);
#2676=VECTOR('',#9546,1.);
#2677=VECTOR('',#9549,1.);
#2678=VECTOR('',#9550,1.);
#2679=VECTOR('',#9551,1.);
#2680=VECTOR('',#9552,1.);
#2681=VECTOR('',#9555,1.);
#2682=VECTOR('',#9556,1.);
#2683=VECTOR('',#9557,1.);
#2684=VECTOR('',#9560,1.);
#2685=VECTOR('',#9561,1.);
#2686=VECTOR('',#9562,1.);
#2687=VECTOR('',#9563,1.);
#2688=VECTOR('',#9566,1.);
#2689=VECTOR('',#9567,1.);
#2690=VECTOR('',#9568,1.);
#2691=VECTOR('',#9571,1.);
#2692=VECTOR('',#9572,1.);
#2693=VECTOR('',#9573,1.);
#2694=VECTOR('',#9574,1.);
#2695=VECTOR('',#9577,1.);
#2696=VECTOR('',#9578,1.);
#2697=VECTOR('',#9579,1.);
#2698=VECTOR('',#9582,1.);
#2699=VECTOR('',#9583,1.);
#2700=VECTOR('',#9584,1.);
#2701=VECTOR('',#9585,1.);
#2702=VECTOR('',#9588,1.);
#2703=VECTOR('',#9589,1.);
#2704=VECTOR('',#9590,1.);
#2705=VECTOR('',#9593,1.);
#2706=VECTOR('',#9594,1.);
#2707=VECTOR('',#9595,1.);
#2708=VECTOR('',#9596,1.);
#2709=VECTOR('',#9599,1.);
#2710=VECTOR('',#9600,1.);
#2711=VECTOR('',#9601,1.);
#2712=VECTOR('',#9604,1.);
#2713=VECTOR('',#9605,1.);
#2714=VECTOR('',#9606,1.);
#2715=VECTOR('',#9607,1.);
#2716=VECTOR('',#9610,1.);
#2717=VECTOR('',#9611,1.);
#2718=VECTOR('',#9612,1.);
#2719=VECTOR('',#9615,1.);
#2720=VECTOR('',#9616,1.);
#2721=VECTOR('',#9617,1.);
#2722=VECTOR('',#9618,1.);
#2723=VECTOR('',#9621,1.);
#2724=VECTOR('',#9622,1.);
#2725=VECTOR('',#9623,1.);
#2726=VECTOR('',#9626,1.);
#2727=VECTOR('',#9627,1.);
#2728=VECTOR('',#9628,1.);
#2729=VECTOR('',#9629,1.);
#2730=VECTOR('',#9632,1.);
#2731=VECTOR('',#9633,1.);
#2732=VECTOR('',#9634,1.);
#2733=VECTOR('',#9637,1.);
#2734=VECTOR('',#9638,1.);
#2735=VECTOR('',#9639,1.);
#2736=VECTOR('',#9640,1.);
#2737=VECTOR('',#9643,1.);
#2738=VECTOR('',#9644,1.);
#2739=VECTOR('',#9645,1.);
#2740=VECTOR('',#9648,1.);
#2741=VECTOR('',#9649,1.);
#2742=VECTOR('',#9650,1.);
#2743=VECTOR('',#9651,1.);
#2744=VECTOR('',#9654,1.);
#2745=VECTOR('',#9655,1.);
#2746=VECTOR('',#9656,1.);
#2747=VECTOR('',#9659,1.);
#2748=VECTOR('',#9660,1.);
#2749=VECTOR('',#9661,1.);
#2750=VECTOR('',#9662,1.);
#2751=VECTOR('',#9665,1.);
#2752=VECTOR('',#9666,1.);
#2753=VECTOR('',#9667,1.);
#2754=VECTOR('',#9670,1.);
#2755=VECTOR('',#9671,1.);
#2756=VECTOR('',#9672,1.);
#2757=VECTOR('',#9673,1.);
#2758=VECTOR('',#9676,1.);
#2759=VECTOR('',#9677,1.);
#2760=VECTOR('',#9678,1.);
#2761=VECTOR('',#9681,1.);
#2762=VECTOR('',#9682,1.);
#2763=VECTOR('',#9683,1.);
#2764=VECTOR('',#9684,1.);
#2765=VECTOR('',#9687,1.);
#2766=VECTOR('',#9688,1.);
#2767=VECTOR('',#9689,1.);
#2768=VECTOR('',#9692,1.);
#2769=VECTOR('',#9693,1.);
#2770=VECTOR('',#9694,1.);
#2771=VECTOR('',#9695,1.);
#2772=VECTOR('',#9698,1.);
#2773=VECTOR('',#9699,1.);
#2774=VECTOR('',#9700,1.);
#2775=VECTOR('',#9703,1.);
#2776=VECTOR('',#9704,1.);
#2777=VECTOR('',#9705,1.);
#2778=VECTOR('',#9706,1.);
#2779=VECTOR('',#9709,1.);
#2780=VECTOR('',#9710,1.);
#2781=VECTOR('',#9711,1.);
#2782=VECTOR('',#9714,1.);
#2783=VECTOR('',#9715,1.);
#2784=VECTOR('',#9716,1.);
#2785=VECTOR('',#9717,1.);
#2786=VECTOR('',#9720,1.);
#2787=VECTOR('',#9721,1.);
#2788=VECTOR('',#9722,1.);
#2789=VECTOR('',#9725,1.);
#2790=VECTOR('',#9726,1.);
#2791=VECTOR('',#9727,1.);
#2792=VECTOR('',#9728,1.);
#2793=VECTOR('',#9731,1.);
#2794=VECTOR('',#9732,1.);
#2795=VECTOR('',#9733,1.);
#2796=VECTOR('',#9736,1.);
#2797=VECTOR('',#9737,1.);
#2798=VECTOR('',#9738,1.);
#2799=VECTOR('',#9739,1.);
#2800=VECTOR('',#9742,1.);
#2801=VECTOR('',#9743,1.);
#2802=VECTOR('',#9744,1.);
#2803=VECTOR('',#9747,1.);
#2804=VECTOR('',#9748,1.);
#2805=VECTOR('',#9749,1.);
#2806=VECTOR('',#9750,1.);
#2807=VECTOR('',#9753,1.);
#2808=VECTOR('',#9754,1.);
#2809=VECTOR('',#9755,1.);
#2810=VECTOR('',#9758,1.);
#2811=VECTOR('',#9759,1.);
#2812=VECTOR('',#9760,1.);
#2813=VECTOR('',#9761,1.);
#2814=VECTOR('',#9764,1.);
#2815=VECTOR('',#9765,1.);
#2816=VECTOR('',#9766,1.);
#2817=VECTOR('',#9769,1.);
#2818=VECTOR('',#9770,1.);
#2819=VECTOR('',#9771,1.);
#2820=VECTOR('',#9772,1.);
#2821=VECTOR('',#9775,1.);
#2822=VECTOR('',#9776,1.);
#2823=VECTOR('',#9777,1.);
#2824=VECTOR('',#9780,1.);
#2825=VECTOR('',#9781,1.);
#2826=VECTOR('',#9782,1.);
#2827=VECTOR('',#9783,1.);
#2828=VECTOR('',#9786,1.);
#2829=VECTOR('',#9787,1.);
#2830=VECTOR('',#9788,1.);
#2831=VECTOR('',#9791,1.);
#2832=VECTOR('',#9792,1.);
#2833=VECTOR('',#9793,1.);
#2834=VECTOR('',#9794,1.);
#2835=VECTOR('',#9797,1.);
#2836=VECTOR('',#9798,1.);
#2837=VECTOR('',#9799,1.);
#2838=VECTOR('',#9802,1.);
#2839=VECTOR('',#9803,1.);
#2840=VECTOR('',#9804,1.);
#2841=VECTOR('',#9805,1.);
#2842=VECTOR('',#9808,1.);
#2843=VECTOR('',#9809,1.);
#2844=VECTOR('',#9810,1.);
#2845=VECTOR('',#9813,1.);
#2846=VECTOR('',#9814,1.);
#2847=VECTOR('',#9815,1.);
#2848=VECTOR('',#9816,1.);
#2849=VECTOR('',#9819,1.);
#2850=VECTOR('',#9820,1.);
#2851=VECTOR('',#9821,1.);
#2852=VECTOR('',#9824,1.);
#2853=VECTOR('',#9825,1.);
#2854=VECTOR('',#9826,1.);
#2855=VECTOR('',#9827,1.);
#2856=VECTOR('',#9830,1.);
#2857=VECTOR('',#9831,1.);
#2858=VECTOR('',#9832,1.);
#2859=VECTOR('',#9835,1.);
#2860=VECTOR('',#9836,1.);
#2861=VECTOR('',#9837,1.);
#2862=VECTOR('',#9838,1.);
#2863=VECTOR('',#9841,1.);
#2864=VECTOR('',#9842,1.);
#2865=VECTOR('',#9843,1.);
#2866=VECTOR('',#9846,1.);
#2867=VECTOR('',#9847,1.);
#2868=VECTOR('',#9848,1.);
#2869=VECTOR('',#9849,1.);
#2870=VECTOR('',#9852,1.);
#2871=VECTOR('',#9853,1.);
#2872=VECTOR('',#9854,1.);
#2873=VECTOR('',#9857,1.);
#2874=VECTOR('',#9858,1.);
#2875=VECTOR('',#9859,1.);
#2876=VECTOR('',#9860,1.);
#2877=VECTOR('',#9863,1.);
#2878=VECTOR('',#9864,1.);
#2879=VECTOR('',#9865,1.);
#2880=VECTOR('',#9868,1.);
#2881=VECTOR('',#9869,1.);
#2882=VECTOR('',#9870,1.);
#2883=VECTOR('',#9871,1.);
#2884=VECTOR('',#9874,1.);
#2885=VECTOR('',#9875,1.);
#2886=VECTOR('',#9876,1.);
#2887=VECTOR('',#9879,1.);
#2888=VECTOR('',#9880,1.);
#2889=VECTOR('',#9881,1.);
#2890=VECTOR('',#9882,1.);
#2891=VECTOR('',#9885,1.);
#2892=VECTOR('',#9886,1.);
#2893=VECTOR('',#9887,1.);
#2894=VECTOR('',#9890,1.);
#2895=VECTOR('',#9891,1.);
#2896=VECTOR('',#9892,1.);
#2897=VECTOR('',#9893,1.);
#2898=VECTOR('',#9896,1.);
#2899=VECTOR('',#9897,1.);
#2900=VECTOR('',#9898,1.);
#2901=VECTOR('',#9901,1.);
#2902=VECTOR('',#9902,1.);
#2903=VECTOR('',#9903,1.);
#2904=VECTOR('',#9904,1.);
#2905=VECTOR('',#9907,1.);
#2906=VECTOR('',#9908,1.);
#2907=VECTOR('',#9909,1.);
#2908=VECTOR('',#9912,1.);
#2909=VECTOR('',#9913,1.);
#2910=VECTOR('',#9914,1.);
#2911=VECTOR('',#9915,1.);
#2912=VECTOR('',#9918,1.);
#2913=VECTOR('',#9919,1.);
#2914=VECTOR('',#9920,1.);
#2915=VECTOR('',#9923,1.);
#2916=VECTOR('',#9924,1.);
#2917=VECTOR('',#9925,1.);
#2918=VECTOR('',#9926,1.);
#2919=VECTOR('',#9929,1.);
#2920=VECTOR('',#9930,1.);
#2921=VECTOR('',#9931,1.);
#2922=VECTOR('',#9934,1.);
#2923=VECTOR('',#9935,1.);
#2924=VECTOR('',#9936,1.);
#2925=VECTOR('',#9937,1.);
#2926=VECTOR('',#9940,1.);
#2927=VECTOR('',#9941,1.);
#2928=VECTOR('',#9942,1.);
#2929=VECTOR('',#9945,1.);
#2930=VECTOR('',#9946,1.);
#2931=VECTOR('',#9947,1.);
#2932=VECTOR('',#9948,1.);
#2933=VECTOR('',#9949,1.);
#2934=VECTOR('',#9952,1.);
#2935=VECTOR('',#9953,1.);
#2936=VECTOR('',#9956,1.);
#2937=VECTOR('',#9957,1.);
#2938=VECTOR('',#9960,1.);
#2939=VECTOR('',#9961,1.);
#2940=VECTOR('',#9964,1.);
#2941=VECTOR('',#9965,1.);
#2942=VECTOR('',#9968,1.);
#2943=VECTOR('',#9969,1.);
#2944=VECTOR('',#9972,1.);
#2945=VECTOR('',#9973,1.);
#2946=VECTOR('',#9976,1.);
#2947=VECTOR('',#9977,1.);
#2948=VECTOR('',#9980,1.);
#2949=VECTOR('',#9981,1.);
#2950=VECTOR('',#9984,1.);
#2951=VECTOR('',#9985,1.);
#2952=VECTOR('',#9988,1.);
#2953=VECTOR('',#9989,1.);
#2954=VECTOR('',#9992,1.);
#2955=VECTOR('',#9993,1.);
#2956=VECTOR('',#9996,1.);
#2957=VECTOR('',#9997,1.);
#2958=VECTOR('',#10000,1.);
#2959=VECTOR('',#10001,1.);
#2960=VECTOR('',#10004,1.);
#2961=VECTOR('',#10005,1.);
#2962=VECTOR('',#10008,1.);
#2963=VECTOR('',#10009,1.);
#2964=VECTOR('',#10012,1.);
#2965=VECTOR('',#10013,1.);
#2966=VECTOR('',#10016,1.);
#2967=VECTOR('',#10017,1.);
#2968=VECTOR('',#10020,1.);
#2969=VECTOR('',#10021,1.);
#2970=VECTOR('',#10024,1.);
#2971=VECTOR('',#10025,1.);
#2972=VECTOR('',#10028,1.);
#2973=VECTOR('',#10029,1.);
#2974=VECTOR('',#10032,1.);
#2975=VECTOR('',#10033,1.);
#2976=VECTOR('',#10036,1.);
#2977=VECTOR('',#10037,1.);
#2978=VECTOR('',#10040,1.);
#2979=VECTOR('',#10041,1.);
#2980=VECTOR('',#10044,1.);
#2981=VECTOR('',#10045,1.);
#2982=VECTOR('',#10048,1.);
#2983=VECTOR('',#10049,1.);
#2984=VECTOR('',#10052,1.);
#2985=VECTOR('',#10053,1.);
#2986=VECTOR('',#10056,1.);
#2987=VECTOR('',#10057,1.);
#2988=VECTOR('',#10060,1.);
#2989=VECTOR('',#10061,1.);
#2990=VECTOR('',#10064,1.);
#2991=VECTOR('',#10065,1.);
#2992=VECTOR('',#10066,1.);
#2993=VECTOR('',#10069,1.);
#2994=VECTOR('',#10070,1.);
#2995=VECTOR('',#10073,1.);
#2996=VECTOR('',#10074,1.);
#2997=VECTOR('',#10077,1.);
#2998=VECTOR('',#10078,1.);
#2999=VECTOR('',#10081,1.);
#3000=VECTOR('',#10082,1.);
#3001=VECTOR('',#10085,1.);
#3002=VECTOR('',#10086,1.);
#3003=VECTOR('',#10089,1.);
#3004=VECTOR('',#10090,1.);
#3005=VECTOR('',#10093,1.);
#3006=VECTOR('',#10094,1.);
#3007=VECTOR('',#10097,1.);
#3008=VECTOR('',#10098,1.);
#3009=VECTOR('',#10101,1.);
#3010=VECTOR('',#10102,1.);
#3011=VECTOR('',#10105,1.);
#3012=VECTOR('',#10106,1.);
#3013=VECTOR('',#10107,1.);
#3014=VECTOR('',#10108,1.);
#3015=VECTOR('',#10111,1.);
#3016=VECTOR('',#10112,1.);
#3017=VECTOR('',#10115,1.);
#3018=VECTOR('',#10116,1.);
#3019=VECTOR('',#10117,1.);
#3020=VECTOR('',#10118,1.);
#3021=VECTOR('',#10121,1.);
#3022=VECTOR('',#10122,1.);
#3023=VECTOR('',#10125,1.);
#3024=VECTOR('',#10126,1.);
#3025=VECTOR('',#10129,1.);
#3026=VECTOR('',#10130,1.);
#3027=VECTOR('',#10135,1.);
#3028=VECTOR('',#10136,1.);
#3029=VECTOR('',#10137,1.);
#3030=VECTOR('',#10138,1.);
#3031=VECTOR('',#10139,1.);
#3032=VECTOR('',#10140,1.);
#3033=VECTOR('',#10147,1.);
#3034=VECTOR('',#10150,1.);
#3035=VECTOR('',#10151,1.);
#3036=VECTOR('',#10152,1.);
#3037=VECTOR('',#10155,1.);
#3038=VECTOR('',#10156,1.);
#3039=VECTOR('',#10159,1.);
#3040=VECTOR('',#10160,1.);
#3041=VECTOR('',#10163,1.);
#3042=VECTOR('',#10164,1.);
#3043=VECTOR('',#10167,1.);
#3044=VECTOR('',#10168,1.);
#3045=VECTOR('',#10171,1.);
#3390=CIRCLE('',#8915,0.17);
#3391=CIRCLE('',#8916,0.17);
#3392=CIRCLE('',#8918,0.17);
#3393=CIRCLE('',#8919,0.17);
#3394=CIRCLE('',#8921,0.41);
#3395=CIRCLE('',#8922,0.41);
#3396=CIRCLE('',#9045,1.4);
#3397=CIRCLE('',#9046,1.4);
#3398=CIRCLE('',#9048,1.4);
#3399=CIRCLE('',#9056,1.4);
#3548=VERTEX_POINT('',#11409);
#3549=VERTEX_POINT('',#11411);
#3550=VERTEX_POINT('',#11415);
#3551=VERTEX_POINT('',#11417);
#3552=VERTEX_POINT('',#11421);
#3553=VERTEX_POINT('',#11423);
#3554=VERTEX_POINT('',#11427);
#3555=VERTEX_POINT('',#11428);
#3556=VERTEX_POINT('',#11430);
#3557=VERTEX_POINT('',#11432);
#3558=VERTEX_POINT('',#11436);
#3559=VERTEX_POINT('',#11437);
#3560=VERTEX_POINT('',#11442);
#3561=VERTEX_POINT('',#11443);
#3562=VERTEX_POINT('',#11445);
#3563=VERTEX_POINT('',#11447);
#3564=VERTEX_POINT('',#11451);
#3565=VERTEX_POINT('',#11452);
#3566=VERTEX_POINT('',#11457);
#3567=VERTEX_POINT('',#11458);
#3568=VERTEX_POINT('',#11460);
#3569=VERTEX_POINT('',#11462);
#3570=VERTEX_POINT('',#11466);
#3571=VERTEX_POINT('',#11467);
#3572=VERTEX_POINT('',#11472);
#3573=VERTEX_POINT('',#11473);
#3574=VERTEX_POINT('',#11475);
#3575=VERTEX_POINT('',#11477);
#3576=VERTEX_POINT('',#11481);
#3577=VERTEX_POINT('',#11482);
#3578=VERTEX_POINT('',#11487);
#3579=VERTEX_POINT('',#11488);
#3580=VERTEX_POINT('',#11490);
#3581=VERTEX_POINT('',#11492);
#3582=VERTEX_POINT('',#11496);
#3583=VERTEX_POINT('',#11497);
#3584=VERTEX_POINT('',#11502);
#3585=VERTEX_POINT('',#11503);
#3586=VERTEX_POINT('',#11505);
#3587=VERTEX_POINT('',#11507);
#3588=VERTEX_POINT('',#11511);
#3589=VERTEX_POINT('',#11512);
#3590=VERTEX_POINT('',#11517);
#3591=VERTEX_POINT('',#11518);
#3592=VERTEX_POINT('',#11520);
#3593=VERTEX_POINT('',#11522);
#3594=VERTEX_POINT('',#11526);
#3595=VERTEX_POINT('',#11527);
#3596=VERTEX_POINT('',#11532);
#3597=VERTEX_POINT('',#11533);
#3598=VERTEX_POINT('',#11535);
#3599=VERTEX_POINT('',#11537);
#3600=VERTEX_POINT('',#11541);
#3601=VERTEX_POINT('',#11542);
#3602=VERTEX_POINT('',#11547);
#3603=VERTEX_POINT('',#11548);
#3604=VERTEX_POINT('',#11550);
#3605=VERTEX_POINT('',#11552);
#3606=VERTEX_POINT('',#11556);
#3607=VERTEX_POINT('',#11557);
#3608=VERTEX_POINT('',#11562);
#3609=VERTEX_POINT('',#11563);
#3610=VERTEX_POINT('',#11565);
#3611=VERTEX_POINT('',#11567);
#3612=VERTEX_POINT('',#11571);
#3613=VERTEX_POINT('',#11572);
#3614=VERTEX_POINT('',#11577);
#3615=VERTEX_POINT('',#11578);
#3616=VERTEX_POINT('',#11580);
#3617=VERTEX_POINT('',#11582);
#3618=VERTEX_POINT('',#11586);
#3619=VERTEX_POINT('',#11587);
#3620=VERTEX_POINT('',#11592);
#3621=VERTEX_POINT('',#11593);
#3622=VERTEX_POINT('',#11595);
#3623=VERTEX_POINT('',#11597);
#3624=VERTEX_POINT('',#11601);
#3625=VERTEX_POINT('',#11602);
#3626=VERTEX_POINT('',#11607);
#3627=VERTEX_POINT('',#11608);
#3628=VERTEX_POINT('',#11610);
#3629=VERTEX_POINT('',#11612);
#3630=VERTEX_POINT('',#11616);
#3631=VERTEX_POINT('',#11617);
#3632=VERTEX_POINT('',#11622);
#3633=VERTEX_POINT('',#11623);
#3634=VERTEX_POINT('',#11625);
#3635=VERTEX_POINT('',#11627);
#3636=VERTEX_POINT('',#11631);
#3637=VERTEX_POINT('',#11632);
#3638=VERTEX_POINT('',#11637);
#3639=VERTEX_POINT('',#11638);
#3640=VERTEX_POINT('',#11640);
#3641=VERTEX_POINT('',#11642);
#3642=VERTEX_POINT('',#11646);
#3643=VERTEX_POINT('',#11647);
#3644=VERTEX_POINT('',#11652);
#3645=VERTEX_POINT('',#11653);
#3646=VERTEX_POINT('',#11655);
#3647=VERTEX_POINT('',#11657);
#3648=VERTEX_POINT('',#11661);
#3649=VERTEX_POINT('',#11662);
#3650=VERTEX_POINT('',#11667);
#3651=VERTEX_POINT('',#11668);
#3652=VERTEX_POINT('',#11670);
#3653=VERTEX_POINT('',#11672);
#3654=VERTEX_POINT('',#11676);
#3655=VERTEX_POINT('',#11677);
#3656=VERTEX_POINT('',#11682);
#3657=VERTEX_POINT('',#11683);
#3658=VERTEX_POINT('',#11685);
#3659=VERTEX_POINT('',#11687);
#3660=VERTEX_POINT('',#11691);
#3661=VERTEX_POINT('',#11692);
#3662=VERTEX_POINT('',#11697);
#3663=VERTEX_POINT('',#11698);
#3664=VERTEX_POINT('',#11700);
#3665=VERTEX_POINT('',#11702);
#3666=VERTEX_POINT('',#11706);
#3667=VERTEX_POINT('',#11707);
#3668=VERTEX_POINT('',#11712);
#3669=VERTEX_POINT('',#11713);
#3670=VERTEX_POINT('',#11715);
#3671=VERTEX_POINT('',#11717);
#3672=VERTEX_POINT('',#11721);
#3673=VERTEX_POINT('',#11722);
#3674=VERTEX_POINT('',#11727);
#3675=VERTEX_POINT('',#11728);
#3676=VERTEX_POINT('',#11730);
#3677=VERTEX_POINT('',#11732);
#3678=VERTEX_POINT('',#11736);
#3679=VERTEX_POINT('',#11737);
#3680=VERTEX_POINT('',#11742);
#3681=VERTEX_POINT('',#11743);
#3682=VERTEX_POINT('',#11745);
#3683=VERTEX_POINT('',#11747);
#3684=VERTEX_POINT('',#11751);
#3685=VERTEX_POINT('',#11752);
#3686=VERTEX_POINT('',#11757);
#3687=VERTEX_POINT('',#11758);
#3688=VERTEX_POINT('',#11760);
#3689=VERTEX_POINT('',#11762);
#3690=VERTEX_POINT('',#11766);
#3691=VERTEX_POINT('',#11767);
#3692=VERTEX_POINT('',#11772);
#3693=VERTEX_POINT('',#11773);
#3694=VERTEX_POINT('',#11775);
#3695=VERTEX_POINT('',#11777);
#3696=VERTEX_POINT('',#11781);
#3697=VERTEX_POINT('',#11782);
#3698=VERTEX_POINT('',#11787);
#3699=VERTEX_POINT('',#11788);
#3700=VERTEX_POINT('',#11790);
#3701=VERTEX_POINT('',#11792);
#3702=VERTEX_POINT('',#11796);
#3703=VERTEX_POINT('',#11797);
#3704=VERTEX_POINT('',#11802);
#3705=VERTEX_POINT('',#11803);
#3706=VERTEX_POINT('',#11805);
#3707=VERTEX_POINT('',#11807);
#3708=VERTEX_POINT('',#11811);
#3709=VERTEX_POINT('',#11812);
#3710=VERTEX_POINT('',#11817);
#3711=VERTEX_POINT('',#11818);
#3712=VERTEX_POINT('',#11820);
#3713=VERTEX_POINT('',#11822);
#3714=VERTEX_POINT('',#11826);
#3715=VERTEX_POINT('',#11827);
#3716=VERTEX_POINT('',#11832);
#3717=VERTEX_POINT('',#11833);
#3718=VERTEX_POINT('',#11835);
#3719=VERTEX_POINT('',#11837);
#3720=VERTEX_POINT('',#11841);
#3721=VERTEX_POINT('',#11842);
#3722=VERTEX_POINT('',#11847);
#3723=VERTEX_POINT('',#11848);
#3724=VERTEX_POINT('',#11850);
#3725=VERTEX_POINT('',#11852);
#3726=VERTEX_POINT('',#11856);
#3727=VERTEX_POINT('',#11857);
#3728=VERTEX_POINT('',#11862);
#3729=VERTEX_POINT('',#11863);
#3730=VERTEX_POINT('',#11865);
#3731=VERTEX_POINT('',#11867);
#3732=VERTEX_POINT('',#11871);
#3733=VERTEX_POINT('',#11872);
#3734=VERTEX_POINT('',#11877);
#3735=VERTEX_POINT('',#11878);
#3736=VERTEX_POINT('',#11880);
#3737=VERTEX_POINT('',#11882);
#3738=VERTEX_POINT('',#11886);
#3739=VERTEX_POINT('',#11887);
#3740=VERTEX_POINT('',#11892);
#3741=VERTEX_POINT('',#11893);
#3742=VERTEX_POINT('',#11895);
#3743=VERTEX_POINT('',#11897);
#3744=VERTEX_POINT('',#11901);
#3745=VERTEX_POINT('',#11902);
#3746=VERTEX_POINT('',#11907);
#3747=VERTEX_POINT('',#11908);
#3748=VERTEX_POINT('',#11910);
#3749=VERTEX_POINT('',#11912);
#3750=VERTEX_POINT('',#11916);
#3751=VERTEX_POINT('',#11917);
#3752=VERTEX_POINT('',#11922);
#3753=VERTEX_POINT('',#11923);
#3754=VERTEX_POINT('',#11925);
#3755=VERTEX_POINT('',#11927);
#3756=VERTEX_POINT('',#11931);
#3757=VERTEX_POINT('',#11932);
#3758=VERTEX_POINT('',#11937);
#3759=VERTEX_POINT('',#11938);
#3760=VERTEX_POINT('',#11940);
#3761=VERTEX_POINT('',#11942);
#3762=VERTEX_POINT('',#11946);
#3763=VERTEX_POINT('',#11947);
#3764=VERTEX_POINT('',#11952);
#3765=VERTEX_POINT('',#11953);
#3766=VERTEX_POINT('',#11955);
#3767=VERTEX_POINT('',#11957);
#3768=VERTEX_POINT('',#11961);
#3769=VERTEX_POINT('',#11962);
#3770=VERTEX_POINT('',#11967);
#3771=VERTEX_POINT('',#11968);
#3772=VERTEX_POINT('',#11970);
#3773=VERTEX_POINT('',#11972);
#3774=VERTEX_POINT('',#11976);
#3775=VERTEX_POINT('',#11977);
#3776=VERTEX_POINT('',#11982);
#3777=VERTEX_POINT('',#11983);
#3778=VERTEX_POINT('',#11985);
#3779=VERTEX_POINT('',#11987);
#3780=VERTEX_POINT('',#11991);
#3781=VERTEX_POINT('',#11992);
#3782=VERTEX_POINT('',#11997);
#3783=VERTEX_POINT('',#11999);
#3784=VERTEX_POINT('',#12001);
#3785=VERTEX_POINT('',#12003);
#3786=VERTEX_POINT('',#12091);
#3787=VERTEX_POINT('',#12093);
#3788=VERTEX_POINT('',#12124);
#3789=VERTEX_POINT('',#12126);
#3790=VERTEX_POINT('',#12128);
#3791=VERTEX_POINT('',#12132);
#3792=VERTEX_POINT('',#12136);
#3793=VERTEX_POINT('',#12137);
#3794=VERTEX_POINT('',#12139);
#3795=VERTEX_POINT('',#12141);
#3796=VERTEX_POINT('',#12145);
#3797=VERTEX_POINT('',#12149);
#3798=VERTEX_POINT('',#12156);
#3799=VERTEX_POINT('',#12158);
#3800=VERTEX_POINT('',#12160);
#3801=VERTEX_POINT('',#12162);
#3802=VERTEX_POINT('',#12164);
#3803=VERTEX_POINT('',#12166);
#3804=VERTEX_POINT('',#12168);
#3805=VERTEX_POINT('',#12172);
#3806=VERTEX_POINT('',#12176);
#3807=VERTEX_POINT('',#12178);
#3808=VERTEX_POINT('',#12182);
#3809=VERTEX_POINT('',#12186);
#3810=VERTEX_POINT('',#12190);
#3811=VERTEX_POINT('',#12194);
#4376=EDGE_CURVE('',#3548,#3548,#3390,.T.);
#4377=EDGE_CURVE('',#3548,#3549,#1930,.T.);
#4378=EDGE_CURVE('',#3549,#3549,#3391,.T.);
#4379=EDGE_CURVE('',#3550,#3550,#3392,.T.);
#4380=EDGE_CURVE('',#3550,#3551,#1931,.T.);
#4381=EDGE_CURVE('',#3551,#3551,#3393,.T.);
#4382=EDGE_CURVE('',#3552,#3552,#3394,.T.);
#4383=EDGE_CURVE('',#3552,#3553,#1932,.T.);
#4384=EDGE_CURVE('',#3553,#3553,#3395,.T.);
#4385=EDGE_CURVE('',#3554,#3555,#1933,.T.);
#4386=EDGE_CURVE('',#3556,#3554,#1934,.T.);
#4387=EDGE_CURVE('',#3556,#3557,#1935,.T.);
#4388=EDGE_CURVE('',#3555,#3557,#1936,.T.);
#4389=EDGE_CURVE('',#3558,#3559,#1937,.T.);
#4390=EDGE_CURVE('',#3557,#3558,#1938,.T.);
#4391=EDGE_CURVE('',#3559,#3556,#1939,.T.);
#4392=EDGE_CURVE('',#3560,#3561,#1940,.T.);
#4393=EDGE_CURVE('',#3562,#3560,#1941,.T.);
#4394=EDGE_CURVE('',#3562,#3563,#1942,.T.);
#4395=EDGE_CURVE('',#3561,#3563,#1943,.T.);
#4396=EDGE_CURVE('',#3564,#3565,#1944,.T.);
#4397=EDGE_CURVE('',#3563,#3564,#1945,.T.);
#4398=EDGE_CURVE('',#3565,#3562,#1946,.T.);
#4399=EDGE_CURVE('',#3566,#3567,#1947,.T.);
#4400=EDGE_CURVE('',#3568,#3566,#1948,.T.);
#4401=EDGE_CURVE('',#3568,#3569,#1949,.T.);
#4402=EDGE_CURVE('',#3567,#3569,#1950,.T.);
#4403=EDGE_CURVE('',#3570,#3571,#1951,.T.);
#4404=EDGE_CURVE('',#3569,#3570,#1952,.T.);
#4405=EDGE_CURVE('',#3571,#3568,#1953,.T.);
#4406=EDGE_CURVE('',#3572,#3573,#1954,.T.);
#4407=EDGE_CURVE('',#3574,#3572,#1955,.T.);
#4408=EDGE_CURVE('',#3574,#3575,#1956,.T.);
#4409=EDGE_CURVE('',#3573,#3575,#1957,.T.);
#4410=EDGE_CURVE('',#3576,#3577,#1958,.T.);
#4411=EDGE_CURVE('',#3575,#3576,#1959,.T.);
#4412=EDGE_CURVE('',#3577,#3574,#1960,.T.);
#4413=EDGE_CURVE('',#3578,#3579,#1961,.T.);
#4414=EDGE_CURVE('',#3580,#3578,#1962,.T.);
#4415=EDGE_CURVE('',#3580,#3581,#1963,.T.);
#4416=EDGE_CURVE('',#3579,#3581,#1964,.T.);
#4417=EDGE_CURVE('',#3582,#3583,#1965,.T.);
#4418=EDGE_CURVE('',#3581,#3582,#1966,.T.);
#4419=EDGE_CURVE('',#3583,#3580,#1967,.T.);
#4420=EDGE_CURVE('',#3584,#3585,#1968,.T.);
#4421=EDGE_CURVE('',#3586,#3584,#1969,.T.);
#4422=EDGE_CURVE('',#3586,#3587,#1970,.T.);
#4423=EDGE_CURVE('',#3585,#3587,#1971,.T.);
#4424=EDGE_CURVE('',#3588,#3589,#1972,.T.);
#4425=EDGE_CURVE('',#3587,#3588,#1973,.T.);
#4426=EDGE_CURVE('',#3589,#3586,#1974,.T.);
#4427=EDGE_CURVE('',#3590,#3591,#1975,.T.);
#4428=EDGE_CURVE('',#3592,#3590,#1976,.T.);
#4429=EDGE_CURVE('',#3592,#3593,#1977,.T.);
#4430=EDGE_CURVE('',#3591,#3593,#1978,.T.);
#4431=EDGE_CURVE('',#3594,#3595,#1979,.T.);
#4432=EDGE_CURVE('',#3593,#3594,#1980,.T.);
#4433=EDGE_CURVE('',#3595,#3592,#1981,.T.);
#4434=EDGE_CURVE('',#3596,#3597,#1982,.T.);
#4435=EDGE_CURVE('',#3598,#3596,#1983,.T.);
#4436=EDGE_CURVE('',#3598,#3599,#1984,.T.);
#4437=EDGE_CURVE('',#3597,#3599,#1985,.T.);
#4438=EDGE_CURVE('',#3600,#3601,#1986,.T.);
#4439=EDGE_CURVE('',#3599,#3600,#1987,.T.);
#4440=EDGE_CURVE('',#3601,#3598,#1988,.T.);
#4441=EDGE_CURVE('',#3602,#3603,#1989,.T.);
#4442=EDGE_CURVE('',#3604,#3602,#1990,.T.);
#4443=EDGE_CURVE('',#3604,#3605,#1991,.T.);
#4444=EDGE_CURVE('',#3603,#3605,#1992,.T.);
#4445=EDGE_CURVE('',#3606,#3607,#1993,.T.);
#4446=EDGE_CURVE('',#3605,#3606,#1994,.T.);
#4447=EDGE_CURVE('',#3607,#3604,#1995,.T.);
#4448=EDGE_CURVE('',#3608,#3609,#1996,.T.);
#4449=EDGE_CURVE('',#3610,#3608,#1997,.T.);
#4450=EDGE_CURVE('',#3610,#3611,#1998,.T.);
#4451=EDGE_CURVE('',#3609,#3611,#1999,.T.);
#4452=EDGE_CURVE('',#3612,#3613,#2000,.T.);
#4453=EDGE_CURVE('',#3611,#3612,#2001,.T.);
#4454=EDGE_CURVE('',#3613,#3610,#2002,.T.);
#4455=EDGE_CURVE('',#3614,#3615,#2003,.T.);
#4456=EDGE_CURVE('',#3616,#3614,#2004,.T.);
#4457=EDGE_CURVE('',#3616,#3617,#2005,.T.);
#4458=EDGE_CURVE('',#3615,#3617,#2006,.T.);
#4459=EDGE_CURVE('',#3618,#3619,#2007,.T.);
#4460=EDGE_CURVE('',#3617,#3618,#2008,.T.);
#4461=EDGE_CURVE('',#3619,#3616,#2009,.T.);
#4462=EDGE_CURVE('',#3620,#3621,#2010,.T.);
#4463=EDGE_CURVE('',#3622,#3620,#2011,.T.);
#4464=EDGE_CURVE('',#3622,#3623,#2012,.T.);
#4465=EDGE_CURVE('',#3621,#3623,#2013,.T.);
#4466=EDGE_CURVE('',#3624,#3625,#2014,.T.);
#4467=EDGE_CURVE('',#3623,#3624,#2015,.T.);
#4468=EDGE_CURVE('',#3625,#3622,#2016,.T.);
#4469=EDGE_CURVE('',#3626,#3627,#2017,.T.);
#4470=EDGE_CURVE('',#3628,#3626,#2018,.T.);
#4471=EDGE_CURVE('',#3628,#3629,#2019,.T.);
#4472=EDGE_CURVE('',#3627,#3629,#2020,.T.);
#4473=EDGE_CURVE('',#3630,#3631,#2021,.T.);
#4474=EDGE_CURVE('',#3629,#3630,#2022,.T.);
#4475=EDGE_CURVE('',#3631,#3628,#2023,.T.);
#4476=EDGE_CURVE('',#3632,#3633,#2024,.T.);
#4477=EDGE_CURVE('',#3634,#3632,#2025,.T.);
#4478=EDGE_CURVE('',#3634,#3635,#2026,.T.);
#4479=EDGE_CURVE('',#3633,#3635,#2027,.T.);
#4480=EDGE_CURVE('',#3636,#3637,#2028,.T.);
#4481=EDGE_CURVE('',#3635,#3636,#2029,.T.);
#4482=EDGE_CURVE('',#3637,#3634,#2030,.T.);
#4483=EDGE_CURVE('',#3638,#3639,#2031,.T.);
#4484=EDGE_CURVE('',#3640,#3638,#2032,.T.);
#4485=EDGE_CURVE('',#3640,#3641,#2033,.T.);
#4486=EDGE_CURVE('',#3639,#3641,#2034,.T.);
#4487=EDGE_CURVE('',#3642,#3643,#2035,.T.);
#4488=EDGE_CURVE('',#3641,#3642,#2036,.T.);
#4489=EDGE_CURVE('',#3643,#3640,#2037,.T.);
#4490=EDGE_CURVE('',#3644,#3645,#2038,.T.);
#4491=EDGE_CURVE('',#3646,#3644,#2039,.T.);
#4492=EDGE_CURVE('',#3646,#3647,#2040,.T.);
#4493=EDGE_CURVE('',#3645,#3647,#2041,.T.);
#4494=EDGE_CURVE('',#3648,#3649,#2042,.T.);
#4495=EDGE_CURVE('',#3647,#3648,#2043,.T.);
#4496=EDGE_CURVE('',#3649,#3646,#2044,.T.);
#4497=EDGE_CURVE('',#3650,#3651,#2045,.T.);
#4498=EDGE_CURVE('',#3652,#3650,#2046,.T.);
#4499=EDGE_CURVE('',#3652,#3653,#2047,.T.);
#4500=EDGE_CURVE('',#3651,#3653,#2048,.T.);
#4501=EDGE_CURVE('',#3654,#3655,#2049,.T.);
#4502=EDGE_CURVE('',#3653,#3654,#2050,.T.);
#4503=EDGE_CURVE('',#3655,#3652,#2051,.T.);
#4504=EDGE_CURVE('',#3656,#3657,#2052,.T.);
#4505=EDGE_CURVE('',#3658,#3656,#2053,.T.);
#4506=EDGE_CURVE('',#3658,#3659,#2054,.T.);
#4507=EDGE_CURVE('',#3657,#3659,#2055,.T.);
#4508=EDGE_CURVE('',#3660,#3661,#2056,.T.);
#4509=EDGE_CURVE('',#3659,#3660,#2057,.T.);
#4510=EDGE_CURVE('',#3661,#3658,#2058,.T.);
#4511=EDGE_CURVE('',#3662,#3663,#2059,.T.);
#4512=EDGE_CURVE('',#3664,#3662,#2060,.T.);
#4513=EDGE_CURVE('',#3664,#3665,#2061,.T.);
#4514=EDGE_CURVE('',#3663,#3665,#2062,.T.);
#4515=EDGE_CURVE('',#3666,#3667,#2063,.T.);
#4516=EDGE_CURVE('',#3665,#3666,#2064,.T.);
#4517=EDGE_CURVE('',#3667,#3664,#2065,.T.);
#4518=EDGE_CURVE('',#3668,#3669,#2066,.T.);
#4519=EDGE_CURVE('',#3670,#3668,#2067,.T.);
#4520=EDGE_CURVE('',#3670,#3671,#2068,.T.);
#4521=EDGE_CURVE('',#3669,#3671,#2069,.T.);
#4522=EDGE_CURVE('',#3672,#3673,#2070,.T.);
#4523=EDGE_CURVE('',#3671,#3672,#2071,.T.);
#4524=EDGE_CURVE('',#3673,#3670,#2072,.T.);
#4525=EDGE_CURVE('',#3674,#3675,#2073,.T.);
#4526=EDGE_CURVE('',#3676,#3674,#2074,.T.);
#4527=EDGE_CURVE('',#3676,#3677,#2075,.T.);
#4528=EDGE_CURVE('',#3675,#3677,#2076,.T.);
#4529=EDGE_CURVE('',#3678,#3679,#2077,.T.);
#4530=EDGE_CURVE('',#3677,#3678,#2078,.T.);
#4531=EDGE_CURVE('',#3679,#3676,#2079,.T.);
#4532=EDGE_CURVE('',#3680,#3681,#2080,.T.);
#4533=EDGE_CURVE('',#3682,#3680,#2081,.T.);
#4534=EDGE_CURVE('',#3682,#3683,#2082,.T.);
#4535=EDGE_CURVE('',#3681,#3683,#2083,.T.);
#4536=EDGE_CURVE('',#3684,#3685,#2084,.T.);
#4537=EDGE_CURVE('',#3683,#3684,#2085,.T.);
#4538=EDGE_CURVE('',#3685,#3682,#2086,.T.);
#4539=EDGE_CURVE('',#3686,#3687,#2087,.T.);
#4540=EDGE_CURVE('',#3688,#3686,#2088,.T.);
#4541=EDGE_CURVE('',#3688,#3689,#2089,.T.);
#4542=EDGE_CURVE('',#3687,#3689,#2090,.T.);
#4543=EDGE_CURVE('',#3690,#3691,#2091,.T.);
#4544=EDGE_CURVE('',#3689,#3690,#2092,.T.);
#4545=EDGE_CURVE('',#3691,#3688,#2093,.T.);
#4546=EDGE_CURVE('',#3692,#3693,#2094,.T.);
#4547=EDGE_CURVE('',#3694,#3692,#2095,.T.);
#4548=EDGE_CURVE('',#3694,#3695,#2096,.T.);
#4549=EDGE_CURVE('',#3693,#3695,#2097,.T.);
#4550=EDGE_CURVE('',#3696,#3697,#2098,.T.);
#4551=EDGE_CURVE('',#3695,#3696,#2099,.T.);
#4552=EDGE_CURVE('',#3697,#3694,#2100,.T.);
#4553=EDGE_CURVE('',#3698,#3699,#2101,.T.);
#4554=EDGE_CURVE('',#3700,#3698,#2102,.T.);
#4555=EDGE_CURVE('',#3700,#3701,#2103,.T.);
#4556=EDGE_CURVE('',#3699,#3701,#2104,.T.);
#4557=EDGE_CURVE('',#3702,#3703,#2105,.T.);
#4558=EDGE_CURVE('',#3701,#3702,#2106,.T.);
#4559=EDGE_CURVE('',#3703,#3700,#2107,.T.);
#4560=EDGE_CURVE('',#3704,#3705,#2108,.T.);
#4561=EDGE_CURVE('',#3706,#3704,#2109,.T.);
#4562=EDGE_CURVE('',#3706,#3707,#2110,.T.);
#4563=EDGE_CURVE('',#3705,#3707,#2111,.T.);
#4564=EDGE_CURVE('',#3708,#3709,#2112,.T.);
#4565=EDGE_CURVE('',#3707,#3708,#2113,.T.);
#4566=EDGE_CURVE('',#3709,#3706,#2114,.T.);
#4567=EDGE_CURVE('',#3710,#3711,#2115,.T.);
#4568=EDGE_CURVE('',#3712,#3710,#2116,.T.);
#4569=EDGE_CURVE('',#3712,#3713,#2117,.T.);
#4570=EDGE_CURVE('',#3711,#3713,#2118,.T.);
#4571=EDGE_CURVE('',#3714,#3715,#2119,.T.);
#4572=EDGE_CURVE('',#3713,#3714,#2120,.T.);
#4573=EDGE_CURVE('',#3715,#3712,#2121,.T.);
#4574=EDGE_CURVE('',#3716,#3717,#2122,.T.);
#4575=EDGE_CURVE('',#3718,#3716,#2123,.T.);
#4576=EDGE_CURVE('',#3718,#3719,#2124,.T.);
#4577=EDGE_CURVE('',#3717,#3719,#2125,.T.);
#4578=EDGE_CURVE('',#3720,#3721,#2126,.T.);
#4579=EDGE_CURVE('',#3719,#3720,#2127,.T.);
#4580=EDGE_CURVE('',#3721,#3718,#2128,.T.);
#4581=EDGE_CURVE('',#3722,#3723,#2129,.T.);
#4582=EDGE_CURVE('',#3724,#3722,#2130,.T.);
#4583=EDGE_CURVE('',#3724,#3725,#2131,.T.);
#4584=EDGE_CURVE('',#3723,#3725,#2132,.T.);
#4585=EDGE_CURVE('',#3726,#3727,#2133,.T.);
#4586=EDGE_CURVE('',#3725,#3726,#2134,.T.);
#4587=EDGE_CURVE('',#3727,#3724,#2135,.T.);
#4588=EDGE_CURVE('',#3728,#3729,#2136,.T.);
#4589=EDGE_CURVE('',#3730,#3728,#2137,.T.);
#4590=EDGE_CURVE('',#3730,#3731,#2138,.T.);
#4591=EDGE_CURVE('',#3729,#3731,#2139,.T.);
#4592=EDGE_CURVE('',#3732,#3733,#2140,.T.);
#4593=EDGE_CURVE('',#3731,#3732,#2141,.T.);
#4594=EDGE_CURVE('',#3733,#3730,#2142,.T.);
#4595=EDGE_CURVE('',#3734,#3735,#2143,.T.);
#4596=EDGE_CURVE('',#3736,#3734,#2144,.T.);
#4597=EDGE_CURVE('',#3736,#3737,#2145,.T.);
#4598=EDGE_CURVE('',#3735,#3737,#2146,.T.);
#4599=EDGE_CURVE('',#3738,#3739,#2147,.T.);
#4600=EDGE_CURVE('',#3737,#3738,#2148,.T.);
#4601=EDGE_CURVE('',#3739,#3736,#2149,.T.);
#4602=EDGE_CURVE('',#3740,#3741,#2150,.T.);
#4603=EDGE_CURVE('',#3742,#3740,#2151,.T.);
#4604=EDGE_CURVE('',#3742,#3743,#2152,.T.);
#4605=EDGE_CURVE('',#3741,#3743,#2153,.T.);
#4606=EDGE_CURVE('',#3744,#3745,#2154,.T.);
#4607=EDGE_CURVE('',#3743,#3744,#2155,.T.);
#4608=EDGE_CURVE('',#3745,#3742,#2156,.T.);
#4609=EDGE_CURVE('',#3746,#3747,#2157,.T.);
#4610=EDGE_CURVE('',#3748,#3746,#2158,.T.);
#4611=EDGE_CURVE('',#3748,#3749,#2159,.T.);
#4612=EDGE_CURVE('',#3747,#3749,#2160,.T.);
#4613=EDGE_CURVE('',#3750,#3751,#2161,.T.);
#4614=EDGE_CURVE('',#3749,#3750,#2162,.T.);
#4615=EDGE_CURVE('',#3751,#3748,#2163,.T.);
#4616=EDGE_CURVE('',#3752,#3753,#2164,.T.);
#4617=EDGE_CURVE('',#3754,#3752,#2165,.T.);
#4618=EDGE_CURVE('',#3754,#3755,#2166,.T.);
#4619=EDGE_CURVE('',#3753,#3755,#2167,.T.);
#4620=EDGE_CURVE('',#3756,#3757,#2168,.T.);
#4621=EDGE_CURVE('',#3755,#3756,#2169,.T.);
#4622=EDGE_CURVE('',#3757,#3754,#2170,.T.);
#4623=EDGE_CURVE('',#3758,#3759,#2171,.T.);
#4624=EDGE_CURVE('',#3760,#3758,#2172,.T.);
#4625=EDGE_CURVE('',#3760,#3761,#2173,.T.);
#4626=EDGE_CURVE('',#3759,#3761,#2174,.T.);
#4627=EDGE_CURVE('',#3762,#3763,#2175,.T.);
#4628=EDGE_CURVE('',#3761,#3762,#2176,.T.);
#4629=EDGE_CURVE('',#3763,#3760,#2177,.T.);
#4630=EDGE_CURVE('',#3764,#3765,#2178,.T.);
#4631=EDGE_CURVE('',#3766,#3764,#2179,.T.);
#4632=EDGE_CURVE('',#3766,#3767,#2180,.T.);
#4633=EDGE_CURVE('',#3765,#3767,#2181,.T.);
#4634=EDGE_CURVE('',#3768,#3769,#2182,.T.);
#4635=EDGE_CURVE('',#3767,#3768,#2183,.T.);
#4636=EDGE_CURVE('',#3769,#3766,#2184,.T.);
#4637=EDGE_CURVE('',#3770,#3771,#2185,.T.);
#4638=EDGE_CURVE('',#3772,#3770,#2186,.T.);
#4639=EDGE_CURVE('',#3772,#3773,#2187,.T.);
#4640=EDGE_CURVE('',#3771,#3773,#2188,.T.);
#4641=EDGE_CURVE('',#3774,#3775,#2189,.T.);
#4642=EDGE_CURVE('',#3773,#3774,#2190,.T.);
#4643=EDGE_CURVE('',#3775,#3772,#2191,.T.);
#4644=EDGE_CURVE('',#3776,#3777,#2192,.T.);
#4645=EDGE_CURVE('',#3778,#3776,#2193,.T.);
#4646=EDGE_CURVE('',#3778,#3779,#2194,.T.);
#4647=EDGE_CURVE('',#3777,#3779,#2195,.T.);
#4648=EDGE_CURVE('',#3780,#3781,#2196,.T.);
#4649=EDGE_CURVE('',#3779,#3780,#2197,.T.);
#4650=EDGE_CURVE('',#3781,#3778,#2198,.T.);
#4651=EDGE_CURVE('',#3782,#3777,#2199,.T.);
#4652=EDGE_CURVE('',#3782,#3783,#2200,.T.);
#4653=EDGE_CURVE('',#3784,#3783,#2201,.T.);
#4654=EDGE_CURVE('',#3785,#3784,#2202,.T.);
#4655=EDGE_CURVE('',#3776,#3785,#2203,.T.);
#4656=EDGE_CURVE('',#3780,#3555,#2204,.T.);
#4657=EDGE_CURVE('',#3554,#3781,#2205,.T.);
#4658=EDGE_CURVE('',#3774,#3561,#2206,.T.);
#4659=EDGE_CURVE('',#3560,#3775,#2207,.T.);
#4660=EDGE_CURVE('',#3768,#3567,#2208,.T.);
#4661=EDGE_CURVE('',#3566,#3769,#2209,.T.);
#4662=EDGE_CURVE('',#3762,#3573,#2210,.T.);
#4663=EDGE_CURVE('',#3572,#3763,#2211,.T.);
#4664=EDGE_CURVE('',#3756,#3579,#2212,.T.);
#4665=EDGE_CURVE('',#3578,#3757,#2213,.T.);
#4666=EDGE_CURVE('',#3750,#3585,#2214,.T.);
#4667=EDGE_CURVE('',#3584,#3751,#2215,.T.);
#4668=EDGE_CURVE('',#3744,#3591,#2216,.T.);
#4669=EDGE_CURVE('',#3590,#3745,#2217,.T.);
#4670=EDGE_CURVE('',#3738,#3597,#2218,.T.);
#4671=EDGE_CURVE('',#3596,#3739,#2219,.T.);
#4672=EDGE_CURVE('',#3732,#3603,#2220,.T.);
#4673=EDGE_CURVE('',#3602,#3733,#2221,.T.);
#4674=EDGE_CURVE('',#3726,#3717,#2222,.T.);
#4675=EDGE_CURVE('',#3716,#3727,#2223,.T.);
#4676=EDGE_CURVE('',#3720,#3615,#2224,.T.);
#4677=EDGE_CURVE('',#3614,#3721,#2225,.T.);
#4678=EDGE_CURVE('',#3714,#3621,#2226,.T.);
#4679=EDGE_CURVE('',#3620,#3715,#2227,.T.);
#4680=EDGE_CURVE('',#3708,#3627,#2228,.T.);
#4681=EDGE_CURVE('',#3626,#3709,#2229,.T.);
#4682=EDGE_CURVE('',#3702,#3633,#2230,.T.);
#4683=EDGE_CURVE('',#3632,#3703,#2231,.T.);
#4684=EDGE_CURVE('',#3696,#3639,#2232,.T.);
#4685=EDGE_CURVE('',#3638,#3697,#2233,.T.);
#4686=EDGE_CURVE('',#3690,#3645,#2234,.T.);
#4687=EDGE_CURVE('',#3644,#3691,#2235,.T.);
#4688=EDGE_CURVE('',#3684,#3651,#2236,.T.);
#4689=EDGE_CURVE('',#3650,#3685,#2237,.T.);
#4690=EDGE_CURVE('',#3678,#3657,#2238,.T.);
#4691=EDGE_CURVE('',#3656,#3679,#2239,.T.);
#4692=EDGE_CURVE('',#3672,#3663,#2240,.T.);
#4693=EDGE_CURVE('',#3662,#3673,#2241,.T.);
#4694=EDGE_CURVE('',#3666,#3609,#2242,.T.);
#4695=EDGE_CURVE('',#3608,#3667,#2243,.T.);
#4696=EDGE_CURVE('',#3668,#3661,#2244,.T.);
#4697=EDGE_CURVE('',#3660,#3669,#2245,.T.);
#4698=EDGE_CURVE('',#3674,#3655,#2246,.T.);
#4699=EDGE_CURVE('',#3654,#3675,#2247,.T.);
#4700=EDGE_CURVE('',#3680,#3649,#2248,.T.);
#4701=EDGE_CURVE('',#3648,#3681,#2249,.T.);
#4702=EDGE_CURVE('',#3686,#3643,#2250,.T.);
#4703=EDGE_CURVE('',#3642,#3687,#2251,.T.);
#4704=EDGE_CURVE('',#3692,#3637,#2252,.T.);
#4705=EDGE_CURVE('',#3636,#3693,#2253,.T.);
#4706=EDGE_CURVE('',#3698,#3631,#2254,.T.);
#4707=EDGE_CURVE('',#3630,#3699,#2255,.T.);
#4708=EDGE_CURVE('',#3704,#3625,#2256,.T.);
#4709=EDGE_CURVE('',#3624,#3705,#2257,.T.);
#4710=EDGE_CURVE('',#3710,#3619,#2258,.T.);
#4711=EDGE_CURVE('',#3618,#3711,#2259,.T.);
#4712=EDGE_CURVE('',#3786,#3613,#2260,.T.);
#4713=EDGE_CURVE('',#3787,#3786,#2261,.T.);
#4714=EDGE_CURVE('',#3612,#3787,#2262,.T.);
#4715=EDGE_CURVE('',#3722,#3607,#2263,.T.);
#4716=EDGE_CURVE('',#3606,#3723,#2264,.T.);
#4717=EDGE_CURVE('',#3728,#3601,#2265,.T.);
#4718=EDGE_CURVE('',#3600,#3729,#2266,.T.);
#4719=EDGE_CURVE('',#3734,#3595,#2267,.T.);
#4720=EDGE_CURVE('',#3594,#3735,#2268,.T.);
#4721=EDGE_CURVE('',#3740,#3589,#2269,.T.);
#4722=EDGE_CURVE('',#3588,#3741,#2270,.T.);
#4723=EDGE_CURVE('',#3746,#3583,#2271,.T.);
#4724=EDGE_CURVE('',#3582,#3747,#2272,.T.);
#4725=EDGE_CURVE('',#3752,#3577,#2273,.T.);
#4726=EDGE_CURVE('',#3576,#3753,#2274,.T.);
#4727=EDGE_CURVE('',#3758,#3571,#2275,.T.);
#4728=EDGE_CURVE('',#3570,#3759,#2276,.T.);
#4729=EDGE_CURVE('',#3764,#3565,#2277,.T.);
#4730=EDGE_CURVE('',#3564,#3765,#2278,.T.);
#4731=EDGE_CURVE('',#3770,#3559,#2279,.T.);
#4732=EDGE_CURVE('',#3558,#3771,#2280,.T.);
#4733=EDGE_CURVE('',#3787,#3788,#2281,.T.);
#4734=EDGE_CURVE('',#3788,#3789,#2282,.T.);
#4735=EDGE_CURVE('',#3789,#3790,#2283,.T.);
#4736=EDGE_CURVE('',#3790,#3782,#2284,.T.);
#4737=EDGE_CURVE('',#3790,#3791,#2285,.T.);
#4738=EDGE_CURVE('',#3783,#3791,#2286,.T.);
#4739=EDGE_CURVE('',#3792,#3793,#2287,.T.);
#4740=EDGE_CURVE('',#3794,#3792,#2288,.T.);
#4741=EDGE_CURVE('',#3794,#3795,#2289,.T.);
#4742=EDGE_CURVE('',#3793,#3795,#2290,.T.);
#4743=EDGE_CURVE('',#3796,#3786,#2291,.T.);
#4744=EDGE_CURVE('',#3788,#3796,#2292,.T.);
#4745=EDGE_CURVE('',#3797,#3796,#2293,.T.);
#4746=EDGE_CURVE('',#3789,#3797,#2294,.T.);
#4747=EDGE_CURVE('',#3795,#3797,#2295,.T.);
#4748=EDGE_CURVE('',#3791,#3794,#2296,.T.);
#4749=EDGE_CURVE('',#3798,#3792,#3396,.T.);
#4750=EDGE_CURVE('',#3799,#3798,#2297,.T.);
#4751=EDGE_CURVE('',#3800,#3799,#2298,.T.);
#4752=EDGE_CURVE('',#3801,#3800,#2299,.T.);
#4753=EDGE_CURVE('',#3802,#3801,#2300,.T.);
#4754=EDGE_CURVE('',#3803,#3802,#2301,.T.);
#4755=EDGE_CURVE('',#3804,#3803,#2302,.T.);
#4756=EDGE_CURVE('',#3784,#3804,#3397,.T.);
#4757=EDGE_CURVE('',#3805,#3793,#3398,.T.);
#4758=EDGE_CURVE('',#3805,#3798,#2303,.T.);
#4759=EDGE_CURVE('',#3804,#3806,#2304,.T.);
#4760=EDGE_CURVE('',#3803,#3807,#2305,.T.);
#4761=EDGE_CURVE('',#3806,#3807,#2306,.T.);
#4762=EDGE_CURVE('',#3808,#3805,#2307,.T.);
#4763=EDGE_CURVE('',#3799,#3808,#2308,.T.);
#4764=EDGE_CURVE('',#3809,#3808,#2309,.T.);
#4765=EDGE_CURVE('',#3800,#3809,#2310,.T.);
#4766=EDGE_CURVE('',#3810,#3809,#2311,.T.);
#4767=EDGE_CURVE('',#3801,#3810,#2312,.T.);
#4768=EDGE_CURVE('',#3811,#3810,#2313,.T.);
#4769=EDGE_CURVE('',#3802,#3811,#2314,.T.);
#4770=EDGE_CURVE('',#3807,#3811,#2315,.T.);
#4771=EDGE_CURVE('',#3785,#3806,#3399,.T.);
#5646=ORIENTED_EDGE('',*,*,#4376,.F.);
#5647=ORIENTED_EDGE('',*,*,#4377,.T.);
#5648=ORIENTED_EDGE('',*,*,#4378,.F.);
#5649=ORIENTED_EDGE('',*,*,#4377,.F.);
#5650=ORIENTED_EDGE('',*,*,#4379,.F.);
#5651=ORIENTED_EDGE('',*,*,#4380,.T.);
#5652=ORIENTED_EDGE('',*,*,#4381,.F.);
#5653=ORIENTED_EDGE('',*,*,#4380,.F.);
#5654=ORIENTED_EDGE('',*,*,#4382,.F.);
#5655=ORIENTED_EDGE('',*,*,#4383,.T.);
#5656=ORIENTED_EDGE('',*,*,#4384,.F.);
#5657=ORIENTED_EDGE('',*,*,#4383,.F.);
#5658=ORIENTED_EDGE('',*,*,#4385,.F.);
#5659=ORIENTED_EDGE('',*,*,#4386,.F.);
#5660=ORIENTED_EDGE('',*,*,#4387,.T.);
#5661=ORIENTED_EDGE('',*,*,#4388,.F.);
#5662=ORIENTED_EDGE('',*,*,#4389,.F.);
#5663=ORIENTED_EDGE('',*,*,#4390,.F.);
#5664=ORIENTED_EDGE('',*,*,#4387,.F.);
#5665=ORIENTED_EDGE('',*,*,#4391,.F.);
#5666=ORIENTED_EDGE('',*,*,#4392,.F.);
#5667=ORIENTED_EDGE('',*,*,#4393,.F.);
#5668=ORIENTED_EDGE('',*,*,#4394,.T.);
#5669=ORIENTED_EDGE('',*,*,#4395,.F.);
#5670=ORIENTED_EDGE('',*,*,#4396,.F.);
#5671=ORIENTED_EDGE('',*,*,#4397,.F.);
#5672=ORIENTED_EDGE('',*,*,#4394,.F.);
#5673=ORIENTED_EDGE('',*,*,#4398,.F.);
#5674=ORIENTED_EDGE('',*,*,#4399,.F.);
#5675=ORIENTED_EDGE('',*,*,#4400,.F.);
#5676=ORIENTED_EDGE('',*,*,#4401,.T.);
#5677=ORIENTED_EDGE('',*,*,#4402,.F.);
#5678=ORIENTED_EDGE('',*,*,#4403,.F.);
#5679=ORIENTED_EDGE('',*,*,#4404,.F.);
#5680=ORIENTED_EDGE('',*,*,#4401,.F.);
#5681=ORIENTED_EDGE('',*,*,#4405,.F.);
#5682=ORIENTED_EDGE('',*,*,#4406,.F.);
#5683=ORIENTED_EDGE('',*,*,#4407,.F.);
#5684=ORIENTED_EDGE('',*,*,#4408,.T.);
#5685=ORIENTED_EDGE('',*,*,#4409,.F.);
#5686=ORIENTED_EDGE('',*,*,#4410,.F.);
#5687=ORIENTED_EDGE('',*,*,#4411,.F.);
#5688=ORIENTED_EDGE('',*,*,#4408,.F.);
#5689=ORIENTED_EDGE('',*,*,#4412,.F.);
#5690=ORIENTED_EDGE('',*,*,#4413,.F.);
#5691=ORIENTED_EDGE('',*,*,#4414,.F.);
#5692=ORIENTED_EDGE('',*,*,#4415,.T.);
#5693=ORIENTED_EDGE('',*,*,#4416,.F.);
#5694=ORIENTED_EDGE('',*,*,#4417,.F.);
#5695=ORIENTED_EDGE('',*,*,#4418,.F.);
#5696=ORIENTED_EDGE('',*,*,#4415,.F.);
#5697=ORIENTED_EDGE('',*,*,#4419,.F.);
#5698=ORIENTED_EDGE('',*,*,#4420,.F.);
#5699=ORIENTED_EDGE('',*,*,#4421,.F.);
#5700=ORIENTED_EDGE('',*,*,#4422,.T.);
#5701=ORIENTED_EDGE('',*,*,#4423,.F.);
#5702=ORIENTED_EDGE('',*,*,#4424,.F.);
#5703=ORIENTED_EDGE('',*,*,#4425,.F.);
#5704=ORIENTED_EDGE('',*,*,#4422,.F.);
#5705=ORIENTED_EDGE('',*,*,#4426,.F.);
#5706=ORIENTED_EDGE('',*,*,#4427,.F.);
#5707=ORIENTED_EDGE('',*,*,#4428,.F.);
#5708=ORIENTED_EDGE('',*,*,#4429,.T.);
#5709=ORIENTED_EDGE('',*,*,#4430,.F.);
#5710=ORIENTED_EDGE('',*,*,#4431,.F.);
#5711=ORIENTED_EDGE('',*,*,#4432,.F.);
#5712=ORIENTED_EDGE('',*,*,#4429,.F.);
#5713=ORIENTED_EDGE('',*,*,#4433,.F.);
#5714=ORIENTED_EDGE('',*,*,#4434,.F.);
#5715=ORIENTED_EDGE('',*,*,#4435,.F.);
#5716=ORIENTED_EDGE('',*,*,#4436,.T.);
#5717=ORIENTED_EDGE('',*,*,#4437,.F.);
#5718=ORIENTED_EDGE('',*,*,#4438,.F.);
#5719=ORIENTED_EDGE('',*,*,#4439,.F.);
#5720=ORIENTED_EDGE('',*,*,#4436,.F.);
#5721=ORIENTED_EDGE('',*,*,#4440,.F.);
#5722=ORIENTED_EDGE('',*,*,#4441,.F.);
#5723=ORIENTED_EDGE('',*,*,#4442,.F.);
#5724=ORIENTED_EDGE('',*,*,#4443,.T.);
#5725=ORIENTED_EDGE('',*,*,#4444,.F.);
#5726=ORIENTED_EDGE('',*,*,#4445,.F.);
#5727=ORIENTED_EDGE('',*,*,#4446,.F.);
#5728=ORIENTED_EDGE('',*,*,#4443,.F.);
#5729=ORIENTED_EDGE('',*,*,#4447,.F.);
#5730=ORIENTED_EDGE('',*,*,#4448,.F.);
#5731=ORIENTED_EDGE('',*,*,#4449,.F.);
#5732=ORIENTED_EDGE('',*,*,#4450,.T.);
#5733=ORIENTED_EDGE('',*,*,#4451,.F.);
#5734=ORIENTED_EDGE('',*,*,#4452,.F.);
#5735=ORIENTED_EDGE('',*,*,#4453,.F.);
#5736=ORIENTED_EDGE('',*,*,#4450,.F.);
#5737=ORIENTED_EDGE('',*,*,#4454,.F.);
#5738=ORIENTED_EDGE('',*,*,#4455,.F.);
#5739=ORIENTED_EDGE('',*,*,#4456,.F.);
#5740=ORIENTED_EDGE('',*,*,#4457,.T.);
#5741=ORIENTED_EDGE('',*,*,#4458,.F.);
#5742=ORIENTED_EDGE('',*,*,#4459,.F.);
#5743=ORIENTED_EDGE('',*,*,#4460,.F.);
#5744=ORIENTED_EDGE('',*,*,#4457,.F.);
#5745=ORIENTED_EDGE('',*,*,#4461,.F.);
#5746=ORIENTED_EDGE('',*,*,#4462,.F.);
#5747=ORIENTED_EDGE('',*,*,#4463,.F.);
#5748=ORIENTED_EDGE('',*,*,#4464,.T.);
#5749=ORIENTED_EDGE('',*,*,#4465,.F.);
#5750=ORIENTED_EDGE('',*,*,#4466,.F.);
#5751=ORIENTED_EDGE('',*,*,#4467,.F.);
#5752=ORIENTED_EDGE('',*,*,#4464,.F.);
#5753=ORIENTED_EDGE('',*,*,#4468,.F.);
#5754=ORIENTED_EDGE('',*,*,#4469,.F.);
#5755=ORIENTED_EDGE('',*,*,#4470,.F.);
#5756=ORIENTED_EDGE('',*,*,#4471,.T.);
#5757=ORIENTED_EDGE('',*,*,#4472,.F.);
#5758=ORIENTED_EDGE('',*,*,#4473,.F.);
#5759=ORIENTED_EDGE('',*,*,#4474,.F.);
#5760=ORIENTED_EDGE('',*,*,#4471,.F.);
#5761=ORIENTED_EDGE('',*,*,#4475,.F.);
#5762=ORIENTED_EDGE('',*,*,#4476,.F.);
#5763=ORIENTED_EDGE('',*,*,#4477,.F.);
#5764=ORIENTED_EDGE('',*,*,#4478,.T.);
#5765=ORIENTED_EDGE('',*,*,#4479,.F.);
#5766=ORIENTED_EDGE('',*,*,#4480,.F.);
#5767=ORIENTED_EDGE('',*,*,#4481,.F.);
#5768=ORIENTED_EDGE('',*,*,#4478,.F.);
#5769=ORIENTED_EDGE('',*,*,#4482,.F.);
#5770=ORIENTED_EDGE('',*,*,#4483,.F.);
#5771=ORIENTED_EDGE('',*,*,#4484,.F.);
#5772=ORIENTED_EDGE('',*,*,#4485,.T.);
#5773=ORIENTED_EDGE('',*,*,#4486,.F.);
#5774=ORIENTED_EDGE('',*,*,#4487,.F.);
#5775=ORIENTED_EDGE('',*,*,#4488,.F.);
#5776=ORIENTED_EDGE('',*,*,#4485,.F.);
#5777=ORIENTED_EDGE('',*,*,#4489,.F.);
#5778=ORIENTED_EDGE('',*,*,#4490,.F.);
#5779=ORIENTED_EDGE('',*,*,#4491,.F.);
#5780=ORIENTED_EDGE('',*,*,#4492,.T.);
#5781=ORIENTED_EDGE('',*,*,#4493,.F.);
#5782=ORIENTED_EDGE('',*,*,#4494,.F.);
#5783=ORIENTED_EDGE('',*,*,#4495,.F.);
#5784=ORIENTED_EDGE('',*,*,#4492,.F.);
#5785=ORIENTED_EDGE('',*,*,#4496,.F.);
#5786=ORIENTED_EDGE('',*,*,#4497,.F.);
#5787=ORIENTED_EDGE('',*,*,#4498,.F.);
#5788=ORIENTED_EDGE('',*,*,#4499,.T.);
#5789=ORIENTED_EDGE('',*,*,#4500,.F.);
#5790=ORIENTED_EDGE('',*,*,#4501,.F.);
#5791=ORIENTED_EDGE('',*,*,#4502,.F.);
#5792=ORIENTED_EDGE('',*,*,#4499,.F.);
#5793=ORIENTED_EDGE('',*,*,#4503,.F.);
#5794=ORIENTED_EDGE('',*,*,#4504,.F.);
#5795=ORIENTED_EDGE('',*,*,#4505,.F.);
#5796=ORIENTED_EDGE('',*,*,#4506,.T.);
#5797=ORIENTED_EDGE('',*,*,#4507,.F.);
#5798=ORIENTED_EDGE('',*,*,#4508,.F.);
#5799=ORIENTED_EDGE('',*,*,#4509,.F.);
#5800=ORIENTED_EDGE('',*,*,#4506,.F.);
#5801=ORIENTED_EDGE('',*,*,#4510,.F.);
#5802=ORIENTED_EDGE('',*,*,#4511,.F.);
#5803=ORIENTED_EDGE('',*,*,#4512,.F.);
#5804=ORIENTED_EDGE('',*,*,#4513,.T.);
#5805=ORIENTED_EDGE('',*,*,#4514,.F.);
#5806=ORIENTED_EDGE('',*,*,#4515,.F.);
#5807=ORIENTED_EDGE('',*,*,#4516,.F.);
#5808=ORIENTED_EDGE('',*,*,#4513,.F.);
#5809=ORIENTED_EDGE('',*,*,#4517,.F.);
#5810=ORIENTED_EDGE('',*,*,#4518,.F.);
#5811=ORIENTED_EDGE('',*,*,#4519,.F.);
#5812=ORIENTED_EDGE('',*,*,#4520,.T.);
#5813=ORIENTED_EDGE('',*,*,#4521,.F.);
#5814=ORIENTED_EDGE('',*,*,#4522,.F.);
#5815=ORIENTED_EDGE('',*,*,#4523,.F.);
#5816=ORIENTED_EDGE('',*,*,#4520,.F.);
#5817=ORIENTED_EDGE('',*,*,#4524,.F.);
#5818=ORIENTED_EDGE('',*,*,#4525,.F.);
#5819=ORIENTED_EDGE('',*,*,#4526,.F.);
#5820=ORIENTED_EDGE('',*,*,#4527,.T.);
#5821=ORIENTED_EDGE('',*,*,#4528,.F.);
#5822=ORIENTED_EDGE('',*,*,#4529,.F.);
#5823=ORIENTED_EDGE('',*,*,#4530,.F.);
#5824=ORIENTED_EDGE('',*,*,#4527,.F.);
#5825=ORIENTED_EDGE('',*,*,#4531,.F.);
#5826=ORIENTED_EDGE('',*,*,#4532,.F.);
#5827=ORIENTED_EDGE('',*,*,#4533,.F.);
#5828=ORIENTED_EDGE('',*,*,#4534,.T.);
#5829=ORIENTED_EDGE('',*,*,#4535,.F.);
#5830=ORIENTED_EDGE('',*,*,#4536,.F.);
#5831=ORIENTED_EDGE('',*,*,#4537,.F.);
#5832=ORIENTED_EDGE('',*,*,#4534,.F.);
#5833=ORIENTED_EDGE('',*,*,#4538,.F.);
#5834=ORIENTED_EDGE('',*,*,#4539,.F.);
#5835=ORIENTED_EDGE('',*,*,#4540,.F.);
#5836=ORIENTED_EDGE('',*,*,#4541,.T.);
#5837=ORIENTED_EDGE('',*,*,#4542,.F.);
#5838=ORIENTED_EDGE('',*,*,#4543,.F.);
#5839=ORIENTED_EDGE('',*,*,#4544,.F.);
#5840=ORIENTED_EDGE('',*,*,#4541,.F.);
#5841=ORIENTED_EDGE('',*,*,#4545,.F.);
#5842=ORIENTED_EDGE('',*,*,#4546,.F.);
#5843=ORIENTED_EDGE('',*,*,#4547,.F.);
#5844=ORIENTED_EDGE('',*,*,#4548,.T.);
#5845=ORIENTED_EDGE('',*,*,#4549,.F.);
#5846=ORIENTED_EDGE('',*,*,#4550,.F.);
#5847=ORIENTED_EDGE('',*,*,#4551,.F.);
#5848=ORIENTED_EDGE('',*,*,#4548,.F.);
#5849=ORIENTED_EDGE('',*,*,#4552,.F.);
#5850=ORIENTED_EDGE('',*,*,#4553,.F.);
#5851=ORIENTED_EDGE('',*,*,#4554,.F.);
#5852=ORIENTED_EDGE('',*,*,#4555,.T.);
#5853=ORIENTED_EDGE('',*,*,#4556,.F.);
#5854=ORIENTED_EDGE('',*,*,#4557,.F.);
#5855=ORIENTED_EDGE('',*,*,#4558,.F.);
#5856=ORIENTED_EDGE('',*,*,#4555,.F.);
#5857=ORIENTED_EDGE('',*,*,#4559,.F.);
#5858=ORIENTED_EDGE('',*,*,#4560,.F.);
#5859=ORIENTED_EDGE('',*,*,#4561,.F.);
#5860=ORIENTED_EDGE('',*,*,#4562,.T.);
#5861=ORIENTED_EDGE('',*,*,#4563,.F.);
#5862=ORIENTED_EDGE('',*,*,#4564,.F.);
#5863=ORIENTED_EDGE('',*,*,#4565,.F.);
#5864=ORIENTED_EDGE('',*,*,#4562,.F.);
#5865=ORIENTED_EDGE('',*,*,#4566,.F.);
#5866=ORIENTED_EDGE('',*,*,#4567,.F.);
#5867=ORIENTED_EDGE('',*,*,#4568,.F.);
#5868=ORIENTED_EDGE('',*,*,#4569,.T.);
#5869=ORIENTED_EDGE('',*,*,#4570,.F.);
#5870=ORIENTED_EDGE('',*,*,#4571,.F.);
#5871=ORIENTED_EDGE('',*,*,#4572,.F.);
#5872=ORIENTED_EDGE('',*,*,#4569,.F.);
#5873=ORIENTED_EDGE('',*,*,#4573,.F.);
#5874=ORIENTED_EDGE('',*,*,#4574,.F.);
#5875=ORIENTED_EDGE('',*,*,#4575,.F.);
#5876=ORIENTED_EDGE('',*,*,#4576,.T.);
#5877=ORIENTED_EDGE('',*,*,#4577,.F.);
#5878=ORIENTED_EDGE('',*,*,#4578,.F.);
#5879=ORIENTED_EDGE('',*,*,#4579,.F.);
#5880=ORIENTED_EDGE('',*,*,#4576,.F.);
#5881=ORIENTED_EDGE('',*,*,#4580,.F.);
#5882=ORIENTED_EDGE('',*,*,#4581,.F.);
#5883=ORIENTED_EDGE('',*,*,#4582,.F.);
#5884=ORIENTED_EDGE('',*,*,#4583,.T.);
#5885=ORIENTED_EDGE('',*,*,#4584,.F.);
#5886=ORIENTED_EDGE('',*,*,#4585,.F.);
#5887=ORIENTED_EDGE('',*,*,#4586,.F.);
#5888=ORIENTED_EDGE('',*,*,#4583,.F.);
#5889=ORIENTED_EDGE('',*,*,#4587,.F.);
#5890=ORIENTED_EDGE('',*,*,#4588,.F.);
#5891=ORIENTED_EDGE('',*,*,#4589,.F.);
#5892=ORIENTED_EDGE('',*,*,#4590,.T.);
#5893=ORIENTED_EDGE('',*,*,#4591,.F.);
#5894=ORIENTED_EDGE('',*,*,#4592,.F.);
#5895=ORIENTED_EDGE('',*,*,#4593,.F.);
#5896=ORIENTED_EDGE('',*,*,#4590,.F.);
#5897=ORIENTED_EDGE('',*,*,#4594,.F.);
#5898=ORIENTED_EDGE('',*,*,#4595,.F.);
#5899=ORIENTED_EDGE('',*,*,#4596,.F.);
#5900=ORIENTED_EDGE('',*,*,#4597,.T.);
#5901=ORIENTED_EDGE('',*,*,#4598,.F.);
#5902=ORIENTED_EDGE('',*,*,#4599,.F.);
#5903=ORIENTED_EDGE('',*,*,#4600,.F.);
#5904=ORIENTED_EDGE('',*,*,#4597,.F.);
#5905=ORIENTED_EDGE('',*,*,#4601,.F.);
#5906=ORIENTED_EDGE('',*,*,#4602,.F.);
#5907=ORIENTED_EDGE('',*,*,#4603,.F.);
#5908=ORIENTED_EDGE('',*,*,#4604,.T.);
#5909=ORIENTED_EDGE('',*,*,#4605,.F.);
#5910=ORIENTED_EDGE('',*,*,#4606,.F.);
#5911=ORIENTED_EDGE('',*,*,#4607,.F.);
#5912=ORIENTED_EDGE('',*,*,#4604,.F.);
#5913=ORIENTED_EDGE('',*,*,#4608,.F.);
#5914=ORIENTED_EDGE('',*,*,#4609,.F.);
#5915=ORIENTED_EDGE('',*,*,#4610,.F.);
#5916=ORIENTED_EDGE('',*,*,#4611,.T.);
#5917=ORIENTED_EDGE('',*,*,#4612,.F.);
#5918=ORIENTED_EDGE('',*,*,#4613,.F.);
#5919=ORIENTED_EDGE('',*,*,#4614,.F.);
#5920=ORIENTED_EDGE('',*,*,#4611,.F.);
#5921=ORIENTED_EDGE('',*,*,#4615,.F.);
#5922=ORIENTED_EDGE('',*,*,#4616,.F.);
#5923=ORIENTED_EDGE('',*,*,#4617,.F.);
#5924=ORIENTED_EDGE('',*,*,#4618,.T.);
#5925=ORIENTED_EDGE('',*,*,#4619,.F.);
#5926=ORIENTED_EDGE('',*,*,#4620,.F.);
#5927=ORIENTED_EDGE('',*,*,#4621,.F.);
#5928=ORIENTED_EDGE('',*,*,#4618,.F.);
#5929=ORIENTED_EDGE('',*,*,#4622,.F.);
#5930=ORIENTED_EDGE('',*,*,#4623,.F.);
#5931=ORIENTED_EDGE('',*,*,#4624,.F.);
#5932=ORIENTED_EDGE('',*,*,#4625,.T.);
#5933=ORIENTED_EDGE('',*,*,#4626,.F.);
#5934=ORIENTED_EDGE('',*,*,#4627,.F.);
#5935=ORIENTED_EDGE('',*,*,#4628,.F.);
#5936=ORIENTED_EDGE('',*,*,#4625,.F.);
#5937=ORIENTED_EDGE('',*,*,#4629,.F.);
#5938=ORIENTED_EDGE('',*,*,#4630,.F.);
#5939=ORIENTED_EDGE('',*,*,#4631,.F.);
#5940=ORIENTED_EDGE('',*,*,#4632,.T.);
#5941=ORIENTED_EDGE('',*,*,#4633,.F.);
#5942=ORIENTED_EDGE('',*,*,#4634,.F.);
#5943=ORIENTED_EDGE('',*,*,#4635,.F.);
#5944=ORIENTED_EDGE('',*,*,#4632,.F.);
#5945=ORIENTED_EDGE('',*,*,#4636,.F.);
#5946=ORIENTED_EDGE('',*,*,#4637,.F.);
#5947=ORIENTED_EDGE('',*,*,#4638,.F.);
#5948=ORIENTED_EDGE('',*,*,#4639,.T.);
#5949=ORIENTED_EDGE('',*,*,#4640,.F.);
#5950=ORIENTED_EDGE('',*,*,#4641,.F.);
#5951=ORIENTED_EDGE('',*,*,#4642,.F.);
#5952=ORIENTED_EDGE('',*,*,#4639,.F.);
#5953=ORIENTED_EDGE('',*,*,#4643,.F.);
#5954=ORIENTED_EDGE('',*,*,#4644,.F.);
#5955=ORIENTED_EDGE('',*,*,#4645,.F.);
#5956=ORIENTED_EDGE('',*,*,#4646,.T.);
#5957=ORIENTED_EDGE('',*,*,#4647,.F.);
#5958=ORIENTED_EDGE('',*,*,#4648,.F.);
#5959=ORIENTED_EDGE('',*,*,#4649,.F.);
#5960=ORIENTED_EDGE('',*,*,#4646,.F.);
#5961=ORIENTED_EDGE('',*,*,#4650,.F.);
#5962=ORIENTED_EDGE('',*,*,#4644,.T.);
#5963=ORIENTED_EDGE('',*,*,#4651,.F.);
#5964=ORIENTED_EDGE('',*,*,#4652,.T.);
#5965=ORIENTED_EDGE('',*,*,#4653,.F.);
#5966=ORIENTED_EDGE('',*,*,#4654,.F.);
#5967=ORIENTED_EDGE('',*,*,#4655,.F.);
#5968=ORIENTED_EDGE('',*,*,#4385,.T.);
#5969=ORIENTED_EDGE('',*,*,#4656,.F.);
#5970=ORIENTED_EDGE('',*,*,#4648,.T.);
#5971=ORIENTED_EDGE('',*,*,#4657,.F.);
#5972=ORIENTED_EDGE('',*,*,#4392,.T.);
#5973=ORIENTED_EDGE('',*,*,#4658,.F.);
#5974=ORIENTED_EDGE('',*,*,#4641,.T.);
#5975=ORIENTED_EDGE('',*,*,#4659,.F.);
#5976=ORIENTED_EDGE('',*,*,#4399,.T.);
#5977=ORIENTED_EDGE('',*,*,#4660,.F.);
#5978=ORIENTED_EDGE('',*,*,#4634,.T.);
#5979=ORIENTED_EDGE('',*,*,#4661,.F.);
#5980=ORIENTED_EDGE('',*,*,#4406,.T.);
#5981=ORIENTED_EDGE('',*,*,#4662,.F.);
#5982=ORIENTED_EDGE('',*,*,#4627,.T.);
#5983=ORIENTED_EDGE('',*,*,#4663,.F.);
#5984=ORIENTED_EDGE('',*,*,#4413,.T.);
#5985=ORIENTED_EDGE('',*,*,#4664,.F.);
#5986=ORIENTED_EDGE('',*,*,#4620,.T.);
#5987=ORIENTED_EDGE('',*,*,#4665,.F.);
#5988=ORIENTED_EDGE('',*,*,#4420,.T.);
#5989=ORIENTED_EDGE('',*,*,#4666,.F.);
#5990=ORIENTED_EDGE('',*,*,#4613,.T.);
#5991=ORIENTED_EDGE('',*,*,#4667,.F.);
#5992=ORIENTED_EDGE('',*,*,#4427,.T.);
#5993=ORIENTED_EDGE('',*,*,#4668,.F.);
#5994=ORIENTED_EDGE('',*,*,#4606,.T.);
#5995=ORIENTED_EDGE('',*,*,#4669,.F.);
#5996=ORIENTED_EDGE('',*,*,#4434,.T.);
#5997=ORIENTED_EDGE('',*,*,#4670,.F.);
#5998=ORIENTED_EDGE('',*,*,#4599,.T.);
#5999=ORIENTED_EDGE('',*,*,#4671,.F.);
#6000=ORIENTED_EDGE('',*,*,#4441,.T.);
#6001=ORIENTED_EDGE('',*,*,#4672,.F.);
#6002=ORIENTED_EDGE('',*,*,#4592,.T.);
#6003=ORIENTED_EDGE('',*,*,#4673,.F.);
#6004=ORIENTED_EDGE('',*,*,#4574,.T.);
#6005=ORIENTED_EDGE('',*,*,#4674,.F.);
#6006=ORIENTED_EDGE('',*,*,#4585,.T.);
#6007=ORIENTED_EDGE('',*,*,#4675,.F.);
#6008=ORIENTED_EDGE('',*,*,#4455,.T.);
#6009=ORIENTED_EDGE('',*,*,#4676,.F.);
#6010=ORIENTED_EDGE('',*,*,#4578,.T.);
#6011=ORIENTED_EDGE('',*,*,#4677,.F.);
#6012=ORIENTED_EDGE('',*,*,#4462,.T.);
#6013=ORIENTED_EDGE('',*,*,#4678,.F.);
#6014=ORIENTED_EDGE('',*,*,#4571,.T.);
#6015=ORIENTED_EDGE('',*,*,#4679,.F.);
#6016=ORIENTED_EDGE('',*,*,#4469,.T.);
#6017=ORIENTED_EDGE('',*,*,#4680,.F.);
#6018=ORIENTED_EDGE('',*,*,#4564,.T.);
#6019=ORIENTED_EDGE('',*,*,#4681,.F.);
#6020=ORIENTED_EDGE('',*,*,#4476,.T.);
#6021=ORIENTED_EDGE('',*,*,#4682,.F.);
#6022=ORIENTED_EDGE('',*,*,#4557,.T.);
#6023=ORIENTED_EDGE('',*,*,#4683,.F.);
#6024=ORIENTED_EDGE('',*,*,#4483,.T.);
#6025=ORIENTED_EDGE('',*,*,#4684,.F.);
#6026=ORIENTED_EDGE('',*,*,#4550,.T.);
#6027=ORIENTED_EDGE('',*,*,#4685,.F.);
#6028=ORIENTED_EDGE('',*,*,#4490,.T.);
#6029=ORIENTED_EDGE('',*,*,#4686,.F.);
#6030=ORIENTED_EDGE('',*,*,#4543,.T.);
#6031=ORIENTED_EDGE('',*,*,#4687,.F.);
#6032=ORIENTED_EDGE('',*,*,#4497,.T.);
#6033=ORIENTED_EDGE('',*,*,#4688,.F.);
#6034=ORIENTED_EDGE('',*,*,#4536,.T.);
#6035=ORIENTED_EDGE('',*,*,#4689,.F.);
#6036=ORIENTED_EDGE('',*,*,#4504,.T.);
#6037=ORIENTED_EDGE('',*,*,#4690,.F.);
#6038=ORIENTED_EDGE('',*,*,#4529,.T.);
#6039=ORIENTED_EDGE('',*,*,#4691,.F.);
#6040=ORIENTED_EDGE('',*,*,#4511,.T.);
#6041=ORIENTED_EDGE('',*,*,#4692,.F.);
#6042=ORIENTED_EDGE('',*,*,#4522,.T.);
#6043=ORIENTED_EDGE('',*,*,#4693,.F.);
#6044=ORIENTED_EDGE('',*,*,#4448,.T.);
#6045=ORIENTED_EDGE('',*,*,#4694,.F.);
#6046=ORIENTED_EDGE('',*,*,#4515,.T.);
#6047=ORIENTED_EDGE('',*,*,#4695,.F.);
#6048=ORIENTED_EDGE('',*,*,#4508,.T.);
#6049=ORIENTED_EDGE('',*,*,#4696,.F.);
#6050=ORIENTED_EDGE('',*,*,#4518,.T.);
#6051=ORIENTED_EDGE('',*,*,#4697,.F.);
#6052=ORIENTED_EDGE('',*,*,#4501,.T.);
#6053=ORIENTED_EDGE('',*,*,#4698,.F.);
#6054=ORIENTED_EDGE('',*,*,#4525,.T.);
#6055=ORIENTED_EDGE('',*,*,#4699,.F.);
#6056=ORIENTED_EDGE('',*,*,#4494,.T.);
#6057=ORIENTED_EDGE('',*,*,#4700,.F.);
#6058=ORIENTED_EDGE('',*,*,#4532,.T.);
#6059=ORIENTED_EDGE('',*,*,#4701,.F.);
#6060=ORIENTED_EDGE('',*,*,#4487,.T.);
#6061=ORIENTED_EDGE('',*,*,#4702,.F.);
#6062=ORIENTED_EDGE('',*,*,#4539,.T.);
#6063=ORIENTED_EDGE('',*,*,#4703,.F.);
#6064=ORIENTED_EDGE('',*,*,#4480,.T.);
#6065=ORIENTED_EDGE('',*,*,#4704,.F.);
#6066=ORIENTED_EDGE('',*,*,#4546,.T.);
#6067=ORIENTED_EDGE('',*,*,#4705,.F.);
#6068=ORIENTED_EDGE('',*,*,#4473,.T.);
#6069=ORIENTED_EDGE('',*,*,#4706,.F.);
#6070=ORIENTED_EDGE('',*,*,#4553,.T.);
#6071=ORIENTED_EDGE('',*,*,#4707,.F.);
#6072=ORIENTED_EDGE('',*,*,#4466,.T.);
#6073=ORIENTED_EDGE('',*,*,#4708,.F.);
#6074=ORIENTED_EDGE('',*,*,#4560,.T.);
#6075=ORIENTED_EDGE('',*,*,#4709,.F.);
#6076=ORIENTED_EDGE('',*,*,#4459,.T.);
#6077=ORIENTED_EDGE('',*,*,#4710,.F.);
#6078=ORIENTED_EDGE('',*,*,#4567,.T.);
#6079=ORIENTED_EDGE('',*,*,#4711,.F.);
#6080=ORIENTED_EDGE('',*,*,#4452,.T.);
#6081=ORIENTED_EDGE('',*,*,#4712,.F.);
#6082=ORIENTED_EDGE('',*,*,#4713,.F.);
#6083=ORIENTED_EDGE('',*,*,#4714,.F.);
#6084=ORIENTED_EDGE('',*,*,#4445,.T.);
#6085=ORIENTED_EDGE('',*,*,#4715,.F.);
#6086=ORIENTED_EDGE('',*,*,#4581,.T.);
#6087=ORIENTED_EDGE('',*,*,#4716,.F.);
#6088=ORIENTED_EDGE('',*,*,#4438,.T.);
#6089=ORIENTED_EDGE('',*,*,#4717,.F.);
#6090=ORIENTED_EDGE('',*,*,#4588,.T.);
#6091=ORIENTED_EDGE('',*,*,#4718,.F.);
#6092=ORIENTED_EDGE('',*,*,#4431,.T.);
#6093=ORIENTED_EDGE('',*,*,#4719,.F.);
#6094=ORIENTED_EDGE('',*,*,#4595,.T.);
#6095=ORIENTED_EDGE('',*,*,#4720,.F.);
#6096=ORIENTED_EDGE('',*,*,#4424,.T.);
#6097=ORIENTED_EDGE('',*,*,#4721,.F.);
#6098=ORIENTED_EDGE('',*,*,#4602,.T.);
#6099=ORIENTED_EDGE('',*,*,#4722,.F.);
#6100=ORIENTED_EDGE('',*,*,#4417,.T.);
#6101=ORIENTED_EDGE('',*,*,#4723,.F.);
#6102=ORIENTED_EDGE('',*,*,#4609,.T.);
#6103=ORIENTED_EDGE('',*,*,#4724,.F.);
#6104=ORIENTED_EDGE('',*,*,#4410,.T.);
#6105=ORIENTED_EDGE('',*,*,#4725,.F.);
#6106=ORIENTED_EDGE('',*,*,#4616,.T.);
#6107=ORIENTED_EDGE('',*,*,#4726,.F.);
#6108=ORIENTED_EDGE('',*,*,#4403,.T.);
#6109=ORIENTED_EDGE('',*,*,#4727,.F.);
#6110=ORIENTED_EDGE('',*,*,#4623,.T.);
#6111=ORIENTED_EDGE('',*,*,#4728,.F.);
#6112=ORIENTED_EDGE('',*,*,#4396,.T.);
#6113=ORIENTED_EDGE('',*,*,#4729,.F.);
#6114=ORIENTED_EDGE('',*,*,#4630,.T.);
#6115=ORIENTED_EDGE('',*,*,#4730,.F.);
#6116=ORIENTED_EDGE('',*,*,#4389,.T.);
#6117=ORIENTED_EDGE('',*,*,#4731,.F.);
#6118=ORIENTED_EDGE('',*,*,#4637,.T.);
#6119=ORIENTED_EDGE('',*,*,#4732,.F.);
#6120=ORIENTED_EDGE('',*,*,#4388,.T.);
#6121=ORIENTED_EDGE('',*,*,#4390,.T.);
#6122=ORIENTED_EDGE('',*,*,#4732,.T.);
#6123=ORIENTED_EDGE('',*,*,#4640,.T.);
#6124=ORIENTED_EDGE('',*,*,#4642,.T.);
#6125=ORIENTED_EDGE('',*,*,#4658,.T.);
#6126=ORIENTED_EDGE('',*,*,#4395,.T.);
#6127=ORIENTED_EDGE('',*,*,#4397,.T.);
#6128=ORIENTED_EDGE('',*,*,#4730,.T.);
#6129=ORIENTED_EDGE('',*,*,#4633,.T.);
#6130=ORIENTED_EDGE('',*,*,#4635,.T.);
#6131=ORIENTED_EDGE('',*,*,#4660,.T.);
#6132=ORIENTED_EDGE('',*,*,#4402,.T.);
#6133=ORIENTED_EDGE('',*,*,#4404,.T.);
#6134=ORIENTED_EDGE('',*,*,#4728,.T.);
#6135=ORIENTED_EDGE('',*,*,#4626,.T.);
#6136=ORIENTED_EDGE('',*,*,#4628,.T.);
#6137=ORIENTED_EDGE('',*,*,#4662,.T.);
#6138=ORIENTED_EDGE('',*,*,#4409,.T.);
#6139=ORIENTED_EDGE('',*,*,#4411,.T.);
#6140=ORIENTED_EDGE('',*,*,#4726,.T.);
#6141=ORIENTED_EDGE('',*,*,#4619,.T.);
#6142=ORIENTED_EDGE('',*,*,#4621,.T.);
#6143=ORIENTED_EDGE('',*,*,#4664,.T.);
#6144=ORIENTED_EDGE('',*,*,#4416,.T.);
#6145=ORIENTED_EDGE('',*,*,#4418,.T.);
#6146=ORIENTED_EDGE('',*,*,#4724,.T.);
#6147=ORIENTED_EDGE('',*,*,#4612,.T.);
#6148=ORIENTED_EDGE('',*,*,#4614,.T.);
#6149=ORIENTED_EDGE('',*,*,#4666,.T.);
#6150=ORIENTED_EDGE('',*,*,#4423,.T.);
#6151=ORIENTED_EDGE('',*,*,#4425,.T.);
#6152=ORIENTED_EDGE('',*,*,#4722,.T.);
#6153=ORIENTED_EDGE('',*,*,#4605,.T.);
#6154=ORIENTED_EDGE('',*,*,#4607,.T.);
#6155=ORIENTED_EDGE('',*,*,#4668,.T.);
#6156=ORIENTED_EDGE('',*,*,#4430,.T.);
#6157=ORIENTED_EDGE('',*,*,#4432,.T.);
#6158=ORIENTED_EDGE('',*,*,#4720,.T.);
#6159=ORIENTED_EDGE('',*,*,#4598,.T.);
#6160=ORIENTED_EDGE('',*,*,#4600,.T.);
#6161=ORIENTED_EDGE('',*,*,#4670,.T.);
#6162=ORIENTED_EDGE('',*,*,#4437,.T.);
#6163=ORIENTED_EDGE('',*,*,#4439,.T.);
#6164=ORIENTED_EDGE('',*,*,#4718,.T.);
#6165=ORIENTED_EDGE('',*,*,#4591,.T.);
#6166=ORIENTED_EDGE('',*,*,#4593,.T.);
#6167=ORIENTED_EDGE('',*,*,#4672,.T.);
#6168=ORIENTED_EDGE('',*,*,#4444,.T.);
#6169=ORIENTED_EDGE('',*,*,#4446,.T.);
#6170=ORIENTED_EDGE('',*,*,#4716,.T.);
#6171=ORIENTED_EDGE('',*,*,#4584,.T.);
#6172=ORIENTED_EDGE('',*,*,#4586,.T.);
#6173=ORIENTED_EDGE('',*,*,#4674,.T.);
#6174=ORIENTED_EDGE('',*,*,#4577,.T.);
#6175=ORIENTED_EDGE('',*,*,#4579,.T.);
#6176=ORIENTED_EDGE('',*,*,#4676,.T.);
#6177=ORIENTED_EDGE('',*,*,#4458,.T.);
#6178=ORIENTED_EDGE('',*,*,#4460,.T.);
#6179=ORIENTED_EDGE('',*,*,#4711,.T.);
#6180=ORIENTED_EDGE('',*,*,#4570,.T.);
#6181=ORIENTED_EDGE('',*,*,#4572,.T.);
#6182=ORIENTED_EDGE('',*,*,#4678,.T.);
#6183=ORIENTED_EDGE('',*,*,#4465,.T.);
#6184=ORIENTED_EDGE('',*,*,#4467,.T.);
#6185=ORIENTED_EDGE('',*,*,#4709,.T.);
#6186=ORIENTED_EDGE('',*,*,#4563,.T.);
#6187=ORIENTED_EDGE('',*,*,#4565,.T.);
#6188=ORIENTED_EDGE('',*,*,#4680,.T.);
#6189=ORIENTED_EDGE('',*,*,#4472,.T.);
#6190=ORIENTED_EDGE('',*,*,#4474,.T.);
#6191=ORIENTED_EDGE('',*,*,#4707,.T.);
#6192=ORIENTED_EDGE('',*,*,#4556,.T.);
#6193=ORIENTED_EDGE('',*,*,#4558,.T.);
#6194=ORIENTED_EDGE('',*,*,#4682,.T.);
#6195=ORIENTED_EDGE('',*,*,#4479,.T.);
#6196=ORIENTED_EDGE('',*,*,#4481,.T.);
#6197=ORIENTED_EDGE('',*,*,#4705,.T.);
#6198=ORIENTED_EDGE('',*,*,#4549,.T.);
#6199=ORIENTED_EDGE('',*,*,#4551,.T.);
#6200=ORIENTED_EDGE('',*,*,#4684,.T.);
#6201=ORIENTED_EDGE('',*,*,#4486,.T.);
#6202=ORIENTED_EDGE('',*,*,#4488,.T.);
#6203=ORIENTED_EDGE('',*,*,#4703,.T.);
#6204=ORIENTED_EDGE('',*,*,#4542,.T.);
#6205=ORIENTED_EDGE('',*,*,#4544,.T.);
#6206=ORIENTED_EDGE('',*,*,#4686,.T.);
#6207=ORIENTED_EDGE('',*,*,#4493,.T.);
#6208=ORIENTED_EDGE('',*,*,#4495,.T.);
#6209=ORIENTED_EDGE('',*,*,#4701,.T.);
#6210=ORIENTED_EDGE('',*,*,#4535,.T.);
#6211=ORIENTED_EDGE('',*,*,#4537,.T.);
#6212=ORIENTED_EDGE('',*,*,#4688,.T.);
#6213=ORIENTED_EDGE('',*,*,#4500,.T.);
#6214=ORIENTED_EDGE('',*,*,#4502,.T.);
#6215=ORIENTED_EDGE('',*,*,#4699,.T.);
#6216=ORIENTED_EDGE('',*,*,#4528,.T.);
#6217=ORIENTED_EDGE('',*,*,#4530,.T.);
#6218=ORIENTED_EDGE('',*,*,#4690,.T.);
#6219=ORIENTED_EDGE('',*,*,#4507,.T.);
#6220=ORIENTED_EDGE('',*,*,#4509,.T.);
#6221=ORIENTED_EDGE('',*,*,#4697,.T.);
#6222=ORIENTED_EDGE('',*,*,#4521,.T.);
#6223=ORIENTED_EDGE('',*,*,#4523,.T.);
#6224=ORIENTED_EDGE('',*,*,#4692,.T.);
#6225=ORIENTED_EDGE('',*,*,#4514,.T.);
#6226=ORIENTED_EDGE('',*,*,#4516,.T.);
#6227=ORIENTED_EDGE('',*,*,#4694,.T.);
#6228=ORIENTED_EDGE('',*,*,#4451,.T.);
#6229=ORIENTED_EDGE('',*,*,#4453,.T.);
#6230=ORIENTED_EDGE('',*,*,#4714,.T.);
#6231=ORIENTED_EDGE('',*,*,#4733,.T.);
#6232=ORIENTED_EDGE('',*,*,#4734,.T.);
#6233=ORIENTED_EDGE('',*,*,#4735,.T.);
#6234=ORIENTED_EDGE('',*,*,#4736,.T.);
#6235=ORIENTED_EDGE('',*,*,#4651,.T.);
#6236=ORIENTED_EDGE('',*,*,#4647,.T.);
#6237=ORIENTED_EDGE('',*,*,#4649,.T.);
#6238=ORIENTED_EDGE('',*,*,#4656,.T.);
#6239=ORIENTED_EDGE('',*,*,#4736,.F.);
#6240=ORIENTED_EDGE('',*,*,#4737,.T.);
#6241=ORIENTED_EDGE('',*,*,#4738,.F.);
#6242=ORIENTED_EDGE('',*,*,#4652,.F.);
#6243=ORIENTED_EDGE('',*,*,#4739,.F.);
#6244=ORIENTED_EDGE('',*,*,#4740,.F.);
#6245=ORIENTED_EDGE('',*,*,#4741,.T.);
#6246=ORIENTED_EDGE('',*,*,#4742,.F.);
#6247=ORIENTED_EDGE('',*,*,#4713,.T.);
#6248=ORIENTED_EDGE('',*,*,#4743,.F.);
#6249=ORIENTED_EDGE('',*,*,#4744,.F.);
#6250=ORIENTED_EDGE('',*,*,#4733,.F.);
#6251=ORIENTED_EDGE('',*,*,#4744,.T.);
#6252=ORIENTED_EDGE('',*,*,#4745,.F.);
#6253=ORIENTED_EDGE('',*,*,#4746,.F.);
#6254=ORIENTED_EDGE('',*,*,#4734,.F.);
#6255=ORIENTED_EDGE('',*,*,#4746,.T.);
#6256=ORIENTED_EDGE('',*,*,#4747,.F.);
#6257=ORIENTED_EDGE('',*,*,#4741,.F.);
#6258=ORIENTED_EDGE('',*,*,#4748,.F.);
#6259=ORIENTED_EDGE('',*,*,#4737,.F.);
#6260=ORIENTED_EDGE('',*,*,#4735,.F.);
#6261=ORIENTED_EDGE('',*,*,#4738,.T.);
#6262=ORIENTED_EDGE('',*,*,#4748,.T.);
#6263=ORIENTED_EDGE('',*,*,#4740,.T.);
#6264=ORIENTED_EDGE('',*,*,#4749,.F.);
#6265=ORIENTED_EDGE('',*,*,#4750,.F.);
#6266=ORIENTED_EDGE('',*,*,#4751,.F.);
#6267=ORIENTED_EDGE('',*,*,#4752,.F.);
#6268=ORIENTED_EDGE('',*,*,#4753,.F.);
#6269=ORIENTED_EDGE('',*,*,#4754,.F.);
#6270=ORIENTED_EDGE('',*,*,#4755,.F.);
#6271=ORIENTED_EDGE('',*,*,#4756,.F.);
#6272=ORIENTED_EDGE('',*,*,#4653,.T.);
#6273=ORIENTED_EDGE('',*,*,#4378,.T.);
#6274=ORIENTED_EDGE('',*,*,#4381,.T.);
#6275=ORIENTED_EDGE('',*,*,#4384,.T.);
#6276=ORIENTED_EDGE('',*,*,#4739,.T.);
#6277=ORIENTED_EDGE('',*,*,#4757,.F.);
#6278=ORIENTED_EDGE('',*,*,#4758,.T.);
#6279=ORIENTED_EDGE('',*,*,#4749,.T.);
#6280=ORIENTED_EDGE('',*,*,#4759,.F.);
#6281=ORIENTED_EDGE('',*,*,#4755,.T.);
#6282=ORIENTED_EDGE('',*,*,#4760,.T.);
#6283=ORIENTED_EDGE('',*,*,#4761,.F.);
#6284=ORIENTED_EDGE('',*,*,#4758,.F.);
#6285=ORIENTED_EDGE('',*,*,#4762,.F.);
#6286=ORIENTED_EDGE('',*,*,#4763,.F.);
#6287=ORIENTED_EDGE('',*,*,#4750,.T.);
#6288=ORIENTED_EDGE('',*,*,#4751,.T.);
#6289=ORIENTED_EDGE('',*,*,#4763,.T.);
#6290=ORIENTED_EDGE('',*,*,#4764,.F.);
#6291=ORIENTED_EDGE('',*,*,#4765,.F.);
#6292=ORIENTED_EDGE('',*,*,#4752,.T.);
#6293=ORIENTED_EDGE('',*,*,#4765,.T.);
#6294=ORIENTED_EDGE('',*,*,#4766,.F.);
#6295=ORIENTED_EDGE('',*,*,#4767,.F.);
#6296=ORIENTED_EDGE('',*,*,#4753,.T.);
#6297=ORIENTED_EDGE('',*,*,#4767,.T.);
#6298=ORIENTED_EDGE('',*,*,#4768,.F.);
#6299=ORIENTED_EDGE('',*,*,#4769,.F.);
#6300=ORIENTED_EDGE('',*,*,#4754,.T.);
#6301=ORIENTED_EDGE('',*,*,#4769,.T.);
#6302=ORIENTED_EDGE('',*,*,#4770,.F.);
#6303=ORIENTED_EDGE('',*,*,#4760,.F.);
#6304=ORIENTED_EDGE('',*,*,#4386,.T.);
#6305=ORIENTED_EDGE('',*,*,#4657,.T.);
#6306=ORIENTED_EDGE('',*,*,#4650,.T.);
#6307=ORIENTED_EDGE('',*,*,#4645,.T.);
#6308=ORIENTED_EDGE('',*,*,#4655,.T.);
#6309=ORIENTED_EDGE('',*,*,#4771,.T.);
#6310=ORIENTED_EDGE('',*,*,#4761,.T.);
#6311=ORIENTED_EDGE('',*,*,#4770,.T.);
#6312=ORIENTED_EDGE('',*,*,#4768,.T.);
#6313=ORIENTED_EDGE('',*,*,#4766,.T.);
#6314=ORIENTED_EDGE('',*,*,#4764,.T.);
#6315=ORIENTED_EDGE('',*,*,#4762,.T.);
#6316=ORIENTED_EDGE('',*,*,#4757,.T.);
#6317=ORIENTED_EDGE('',*,*,#4742,.T.);
#6318=ORIENTED_EDGE('',*,*,#4747,.T.);
#6319=ORIENTED_EDGE('',*,*,#4745,.T.);
#6320=ORIENTED_EDGE('',*,*,#4743,.T.);
#6321=ORIENTED_EDGE('',*,*,#4712,.T.);
#6322=ORIENTED_EDGE('',*,*,#4454,.T.);
#6323=ORIENTED_EDGE('',*,*,#4449,.T.);
#6324=ORIENTED_EDGE('',*,*,#4695,.T.);
#6325=ORIENTED_EDGE('',*,*,#4517,.T.);
#6326=ORIENTED_EDGE('',*,*,#4512,.T.);
#6327=ORIENTED_EDGE('',*,*,#4693,.T.);
#6328=ORIENTED_EDGE('',*,*,#4524,.T.);
#6329=ORIENTED_EDGE('',*,*,#4519,.T.);
#6330=ORIENTED_EDGE('',*,*,#4696,.T.);
#6331=ORIENTED_EDGE('',*,*,#4510,.T.);
#6332=ORIENTED_EDGE('',*,*,#4505,.T.);
#6333=ORIENTED_EDGE('',*,*,#4691,.T.);
#6334=ORIENTED_EDGE('',*,*,#4531,.T.);
#6335=ORIENTED_EDGE('',*,*,#4526,.T.);
#6336=ORIENTED_EDGE('',*,*,#4698,.T.);
#6337=ORIENTED_EDGE('',*,*,#4503,.T.);
#6338=ORIENTED_EDGE('',*,*,#4498,.T.);
#6339=ORIENTED_EDGE('',*,*,#4689,.T.);
#6340=ORIENTED_EDGE('',*,*,#4538,.T.);
#6341=ORIENTED_EDGE('',*,*,#4533,.T.);
#6342=ORIENTED_EDGE('',*,*,#4700,.T.);
#6343=ORIENTED_EDGE('',*,*,#4496,.T.);
#6344=ORIENTED_EDGE('',*,*,#4491,.T.);
#6345=ORIENTED_EDGE('',*,*,#4687,.T.);
#6346=ORIENTED_EDGE('',*,*,#4545,.T.);
#6347=ORIENTED_EDGE('',*,*,#4540,.T.);
#6348=ORIENTED_EDGE('',*,*,#4702,.T.);
#6349=ORIENTED_EDGE('',*,*,#4489,.T.);
#6350=ORIENTED_EDGE('',*,*,#4484,.T.);
#6351=ORIENTED_EDGE('',*,*,#4685,.T.);
#6352=ORIENTED_EDGE('',*,*,#4552,.T.);
#6353=ORIENTED_EDGE('',*,*,#4547,.T.);
#6354=ORIENTED_EDGE('',*,*,#4704,.T.);
#6355=ORIENTED_EDGE('',*,*,#4482,.T.);
#6356=ORIENTED_EDGE('',*,*,#4477,.T.);
#6357=ORIENTED_EDGE('',*,*,#4683,.T.);
#6358=ORIENTED_EDGE('',*,*,#4559,.T.);
#6359=ORIENTED_EDGE('',*,*,#4554,.T.);
#6360=ORIENTED_EDGE('',*,*,#4706,.T.);
#6361=ORIENTED_EDGE('',*,*,#4475,.T.);
#6362=ORIENTED_EDGE('',*,*,#4470,.T.);
#6363=ORIENTED_EDGE('',*,*,#4681,.T.);
#6364=ORIENTED_EDGE('',*,*,#4566,.T.);
#6365=ORIENTED_EDGE('',*,*,#4561,.T.);
#6366=ORIENTED_EDGE('',*,*,#4708,.T.);
#6367=ORIENTED_EDGE('',*,*,#4468,.T.);
#6368=ORIENTED_EDGE('',*,*,#4463,.T.);
#6369=ORIENTED_EDGE('',*,*,#4679,.T.);
#6370=ORIENTED_EDGE('',*,*,#4573,.T.);
#6371=ORIENTED_EDGE('',*,*,#4568,.T.);
#6372=ORIENTED_EDGE('',*,*,#4710,.T.);
#6373=ORIENTED_EDGE('',*,*,#4461,.T.);
#6374=ORIENTED_EDGE('',*,*,#4456,.T.);
#6375=ORIENTED_EDGE('',*,*,#4677,.T.);
#6376=ORIENTED_EDGE('',*,*,#4580,.T.);
#6377=ORIENTED_EDGE('',*,*,#4575,.T.);
#6378=ORIENTED_EDGE('',*,*,#4675,.T.);
#6379=ORIENTED_EDGE('',*,*,#4587,.T.);
#6380=ORIENTED_EDGE('',*,*,#4582,.T.);
#6381=ORIENTED_EDGE('',*,*,#4715,.T.);
#6382=ORIENTED_EDGE('',*,*,#4447,.T.);
#6383=ORIENTED_EDGE('',*,*,#4442,.T.);
#6384=ORIENTED_EDGE('',*,*,#4673,.T.);
#6385=ORIENTED_EDGE('',*,*,#4594,.T.);
#6386=ORIENTED_EDGE('',*,*,#4589,.T.);
#6387=ORIENTED_EDGE('',*,*,#4717,.T.);
#6388=ORIENTED_EDGE('',*,*,#4440,.T.);
#6389=ORIENTED_EDGE('',*,*,#4435,.T.);
#6390=ORIENTED_EDGE('',*,*,#4671,.T.);
#6391=ORIENTED_EDGE('',*,*,#4601,.T.);
#6392=ORIENTED_EDGE('',*,*,#4596,.T.);
#6393=ORIENTED_EDGE('',*,*,#4719,.T.);
#6394=ORIENTED_EDGE('',*,*,#4433,.T.);
#6395=ORIENTED_EDGE('',*,*,#4428,.T.);
#6396=ORIENTED_EDGE('',*,*,#4669,.T.);
#6397=ORIENTED_EDGE('',*,*,#4608,.T.);
#6398=ORIENTED_EDGE('',*,*,#4603,.T.);
#6399=ORIENTED_EDGE('',*,*,#4721,.T.);
#6400=ORIENTED_EDGE('',*,*,#4426,.T.);
#6401=ORIENTED_EDGE('',*,*,#4421,.T.);
#6402=ORIENTED_EDGE('',*,*,#4667,.T.);
#6403=ORIENTED_EDGE('',*,*,#4615,.T.);
#6404=ORIENTED_EDGE('',*,*,#4610,.T.);
#6405=ORIENTED_EDGE('',*,*,#4723,.T.);
#6406=ORIENTED_EDGE('',*,*,#4419,.T.);
#6407=ORIENTED_EDGE('',*,*,#4414,.T.);
#6408=ORIENTED_EDGE('',*,*,#4665,.T.);
#6409=ORIENTED_EDGE('',*,*,#4622,.T.);
#6410=ORIENTED_EDGE('',*,*,#4617,.T.);
#6411=ORIENTED_EDGE('',*,*,#4725,.T.);
#6412=ORIENTED_EDGE('',*,*,#4412,.T.);
#6413=ORIENTED_EDGE('',*,*,#4407,.T.);
#6414=ORIENTED_EDGE('',*,*,#4663,.T.);
#6415=ORIENTED_EDGE('',*,*,#4629,.T.);
#6416=ORIENTED_EDGE('',*,*,#4624,.T.);
#6417=ORIENTED_EDGE('',*,*,#4727,.T.);
#6418=ORIENTED_EDGE('',*,*,#4405,.T.);
#6419=ORIENTED_EDGE('',*,*,#4400,.T.);
#6420=ORIENTED_EDGE('',*,*,#4661,.T.);
#6421=ORIENTED_EDGE('',*,*,#4636,.T.);
#6422=ORIENTED_EDGE('',*,*,#4631,.T.);
#6423=ORIENTED_EDGE('',*,*,#4729,.T.);
#6424=ORIENTED_EDGE('',*,*,#4398,.T.);
#6425=ORIENTED_EDGE('',*,*,#4393,.T.);
#6426=ORIENTED_EDGE('',*,*,#4659,.T.);
#6427=ORIENTED_EDGE('',*,*,#4643,.T.);
#6428=ORIENTED_EDGE('',*,*,#4638,.T.);
#6429=ORIENTED_EDGE('',*,*,#4731,.T.);
#6430=ORIENTED_EDGE('',*,*,#4391,.T.);
#6431=ORIENTED_EDGE('',*,*,#4376,.T.);
#6432=ORIENTED_EDGE('',*,*,#4379,.T.);
#6433=ORIENTED_EDGE('',*,*,#4382,.T.);
#6434=ORIENTED_EDGE('',*,*,#4654,.T.);
#6435=ORIENTED_EDGE('',*,*,#4756,.T.);
#6436=ORIENTED_EDGE('',*,*,#4759,.T.);
#6437=ORIENTED_EDGE('',*,*,#4771,.F.);
#8186=CYLINDRICAL_SURFACE('',#8914,0.17);
#8187=CYLINDRICAL_SURFACE('',#8917,0.17);
#8188=CYLINDRICAL_SURFACE('',#8920,0.41);
#8189=CYLINDRICAL_SURFACE('',#9047,1.4);
#8190=CYLINDRICAL_SURFACE('',#9057,1.4);
#8320=ADVANCED_FACE('',(#903),#8186,.F.);
#8321=ADVANCED_FACE('',(#904),#8187,.F.);
#8322=ADVANCED_FACE('',(#905),#8188,.F.);
#8323=ADVANCED_FACE('',(#906),#651,.F.);
#8324=ADVANCED_FACE('',(#907),#652,.F.);
#8325=ADVANCED_FACE('',(#908),#653,.F.);
#8326=ADVANCED_FACE('',(#909),#654,.F.);
#8327=ADVANCED_FACE('',(#910),#655,.F.);
#8328=ADVANCED_FACE('',(#911),#656,.F.);
#8329=ADVANCED_FACE('',(#912),#657,.F.);
#8330=ADVANCED_FACE('',(#913),#658,.F.);
#8331=ADVANCED_FACE('',(#914),#659,.F.);
#8332=ADVANCED_FACE('',(#915),#660,.F.);
#8333=ADVANCED_FACE('',(#916),#661,.F.);
#8334=ADVANCED_FACE('',(#917),#662,.F.);
#8335=ADVANCED_FACE('',(#918),#663,.F.);
#8336=ADVANCED_FACE('',(#919),#664,.F.);
#8337=ADVANCED_FACE('',(#920),#665,.F.);
#8338=ADVANCED_FACE('',(#921),#666,.F.);
#8339=ADVANCED_FACE('',(#922),#667,.F.);
#8340=ADVANCED_FACE('',(#923),#668,.F.);
#8341=ADVANCED_FACE('',(#924),#669,.F.);
#8342=ADVANCED_FACE('',(#925),#670,.F.);
#8343=ADVANCED_FACE('',(#926),#671,.F.);
#8344=ADVANCED_FACE('',(#927),#672,.F.);
#8345=ADVANCED_FACE('',(#928),#673,.F.);
#8346=ADVANCED_FACE('',(#929),#674,.F.);
#8347=ADVANCED_FACE('',(#930),#675,.F.);
#8348=ADVANCED_FACE('',(#931),#676,.F.);
#8349=ADVANCED_FACE('',(#932),#677,.F.);
#8350=ADVANCED_FACE('',(#933),#678,.F.);
#8351=ADVANCED_FACE('',(#934),#679,.F.);
#8352=ADVANCED_FACE('',(#935),#680,.F.);
#8353=ADVANCED_FACE('',(#936),#681,.F.);
#8354=ADVANCED_FACE('',(#937),#682,.F.);
#8355=ADVANCED_FACE('',(#938),#683,.F.);
#8356=ADVANCED_FACE('',(#939),#684,.F.);
#8357=ADVANCED_FACE('',(#940),#685,.F.);
#8358=ADVANCED_FACE('',(#941),#686,.F.);
#8359=ADVANCED_FACE('',(#942),#687,.F.);
#8360=ADVANCED_FACE('',(#943),#688,.F.);
#8361=ADVANCED_FACE('',(#944),#689,.F.);
#8362=ADVANCED_FACE('',(#945),#690,.F.);
#8363=ADVANCED_FACE('',(#946),#691,.F.);
#8364=ADVANCED_FACE('',(#947),#692,.F.);
#8365=ADVANCED_FACE('',(#948),#693,.F.);
#8366=ADVANCED_FACE('',(#949),#694,.F.);
#8367=ADVANCED_FACE('',(#950),#695,.F.);
#8368=ADVANCED_FACE('',(#951),#696,.F.);
#8369=ADVANCED_FACE('',(#952),#697,.F.);
#8370=ADVANCED_FACE('',(#953),#698,.F.);
#8371=ADVANCED_FACE('',(#954),#699,.F.);
#8372=ADVANCED_FACE('',(#955),#700,.F.);
#8373=ADVANCED_FACE('',(#956),#701,.F.);
#8374=ADVANCED_FACE('',(#957),#702,.F.);
#8375=ADVANCED_FACE('',(#958),#703,.F.);
#8376=ADVANCED_FACE('',(#959),#704,.F.);
#8377=ADVANCED_FACE('',(#960),#705,.F.);
#8378=ADVANCED_FACE('',(#961),#706,.F.);
#8379=ADVANCED_FACE('',(#962),#707,.F.);
#8380=ADVANCED_FACE('',(#963),#708,.F.);
#8381=ADVANCED_FACE('',(#964),#709,.F.);
#8382=ADVANCED_FACE('',(#965),#710,.F.);
#8383=ADVANCED_FACE('',(#966),#711,.F.);
#8384=ADVANCED_FACE('',(#967),#712,.F.);
#8385=ADVANCED_FACE('',(#968),#713,.F.);
#8386=ADVANCED_FACE('',(#969),#714,.F.);
#8387=ADVANCED_FACE('',(#970),#715,.F.);
#8388=ADVANCED_FACE('',(#971),#716,.F.);
#8389=ADVANCED_FACE('',(#972),#717,.F.);
#8390=ADVANCED_FACE('',(#973),#718,.F.);
#8391=ADVANCED_FACE('',(#974),#719,.F.);
#8392=ADVANCED_FACE('',(#975),#720,.F.);
#8393=ADVANCED_FACE('',(#976),#721,.F.);
#8394=ADVANCED_FACE('',(#977),#722,.F.);
#8395=ADVANCED_FACE('',(#978),#723,.F.);
#8396=ADVANCED_FACE('',(#979),#724,.F.);
#8397=ADVANCED_FACE('',(#980),#725,.F.);
#8398=ADVANCED_FACE('',(#981),#726,.F.);
#8399=ADVANCED_FACE('',(#982),#727,.T.);
#8400=ADVANCED_FACE('',(#983),#728,.T.);
#8401=ADVANCED_FACE('',(#984),#729,.T.);
#8402=ADVANCED_FACE('',(#985),#730,.T.);
#8403=ADVANCED_FACE('',(#986),#731,.T.);
#8404=ADVANCED_FACE('',(#987),#732,.T.);
#8405=ADVANCED_FACE('',(#988),#733,.T.);
#8406=ADVANCED_FACE('',(#989),#734,.T.);
#8407=ADVANCED_FACE('',(#990),#735,.T.);
#8408=ADVANCED_FACE('',(#991),#736,.T.);
#8409=ADVANCED_FACE('',(#992),#737,.T.);
#8410=ADVANCED_FACE('',(#993),#738,.T.);
#8411=ADVANCED_FACE('',(#994),#739,.T.);
#8412=ADVANCED_FACE('',(#995),#740,.T.);
#8413=ADVANCED_FACE('',(#996),#741,.T.);
#8414=ADVANCED_FACE('',(#997),#742,.T.);
#8415=ADVANCED_FACE('',(#998),#743,.T.);
#8416=ADVANCED_FACE('',(#999),#744,.T.);
#8417=ADVANCED_FACE('',(#1000),#745,.T.);
#8418=ADVANCED_FACE('',(#1001),#746,.T.);
#8419=ADVANCED_FACE('',(#1002),#747,.T.);
#8420=ADVANCED_FACE('',(#1003),#748,.T.);
#8421=ADVANCED_FACE('',(#1004),#749,.T.);
#8422=ADVANCED_FACE('',(#1005),#750,.T.);
#8423=ADVANCED_FACE('',(#1006),#751,.T.);
#8424=ADVANCED_FACE('',(#1007),#752,.T.);
#8425=ADVANCED_FACE('',(#1008),#753,.T.);
#8426=ADVANCED_FACE('',(#1009),#754,.T.);
#8427=ADVANCED_FACE('',(#1010),#755,.T.);
#8428=ADVANCED_FACE('',(#1011),#756,.T.);
#8429=ADVANCED_FACE('',(#1012),#757,.T.);
#8430=ADVANCED_FACE('',(#1013),#758,.T.);
#8431=ADVANCED_FACE('',(#1014),#759,.T.);
#8432=ADVANCED_FACE('',(#1015),#760,.T.);
#8433=ADVANCED_FACE('',(#1016),#761,.T.);
#8434=ADVANCED_FACE('',(#1017),#762,.T.);
#8435=ADVANCED_FACE('',(#1018),#763,.T.);
#8436=ADVANCED_FACE('',(#1019),#764,.T.);
#8437=ADVANCED_FACE('',(#1020),#765,.T.);
#8438=ADVANCED_FACE('',(#1021),#766,.F.);
#8439=ADVANCED_FACE('',(#1022),#767,.T.);
#8440=ADVANCED_FACE('',(#1023),#768,.T.);
#8441=ADVANCED_FACE('',(#1024),#769,.T.);
#8442=ADVANCED_FACE('',(#1025),#770,.T.);
#8443=ADVANCED_FACE('',(#1026),#771,.T.);
#8444=ADVANCED_FACE('',(#1027,#590,#591,#592),#772,.F.);
#8445=ADVANCED_FACE('',(#1028),#8189,.T.);
#8446=ADVANCED_FACE('',(#1029),#773,.T.);
#8447=ADVANCED_FACE('',(#1030),#774,.T.);
#8448=ADVANCED_FACE('',(#1031),#775,.T.);
#8449=ADVANCED_FACE('',(#1032),#776,.T.);
#8450=ADVANCED_FACE('',(#1033),#777,.T.);
#8451=ADVANCED_FACE('',(#1034),#778,.T.);
#8452=ADVANCED_FACE('',(#1035,#593,#594,#595),#779,.T.);
#8453=ADVANCED_FACE('',(#1036),#8190,.T.);
#8803=CLOSED_SHELL('',(#8320,#8321,#8322,#8323,#8324,#8325,#8326,#8327,
#8328,#8329,#8330,#8331,#8332,#8333,#8334,#8335,#8336,#8337,#8338,#8339,
#8340,#8341,#8342,#8343,#8344,#8345,#8346,#8347,#8348,#8349,#8350,#8351,
#8352,#8353,#8354,#8355,#8356,#8357,#8358,#8359,#8360,#8361,#8362,#8363,
#8364,#8365,#8366,#8367,#8368,#8369,#8370,#8371,#8372,#8373,#8374,#8375,
#8376,#8377,#8378,#8379,#8380,#8381,#8382,#8383,#8384,#8385,#8386,#8387,
#8388,#8389,#8390,#8391,#8392,#8393,#8394,#8395,#8396,#8397,#8398,#8399,
#8400,#8401,#8402,#8403,#8404,#8405,#8406,#8407,#8408,#8409,#8410,#8411,
#8412,#8413,#8414,#8415,#8416,#8417,#8418,#8419,#8420,#8421,#8422,#8423,
#8424,#8425,#8426,#8427,#8428,#8429,#8430,#8431,#8432,#8433,#8434,#8435,
#8436,#8437,#8438,#8439,#8440,#8441,#8442,#8443,#8444,#8445,#8446,#8447,
#8448,#8449,#8450,#8451,#8452,#8453));
#8913=AXIS2_PLACEMENT_3D('',#11407,#9502,#9503);
#8914=AXIS2_PLACEMENT_3D('',#11408,#9504,#9505);
#8915=AXIS2_PLACEMENT_3D('',#11410,#9506,#9507);
#8916=AXIS2_PLACEMENT_3D('',#11413,#9509,#9510);
#8917=AXIS2_PLACEMENT_3D('',#11414,#9511,#9512);
#8918=AXIS2_PLACEMENT_3D('',#11416,#9513,#9514);
#8919=AXIS2_PLACEMENT_3D('',#11419,#9516,#9517);
#8920=AXIS2_PLACEMENT_3D('',#11420,#9518,#9519);
#8921=AXIS2_PLACEMENT_3D('',#11422,#9520,#9521);
#8922=AXIS2_PLACEMENT_3D('',#11425,#9523,#9524);
#8923=AXIS2_PLACEMENT_3D('',#11426,#9525,#9526);
#8924=AXIS2_PLACEMENT_3D('',#11435,#9531,#9532);
#8925=AXIS2_PLACEMENT_3D('',#11441,#9536,#9537);
#8926=AXIS2_PLACEMENT_3D('',#11450,#9542,#9543);
#8927=AXIS2_PLACEMENT_3D('',#11456,#9547,#9548);
#8928=AXIS2_PLACEMENT_3D('',#11465,#9553,#9554);
#8929=AXIS2_PLACEMENT_3D('',#11471,#9558,#9559);
#8930=AXIS2_PLACEMENT_3D('',#11480,#9564,#9565);
#8931=AXIS2_PLACEMENT_3D('',#11486,#9569,#9570);
#8932=AXIS2_PLACEMENT_3D('',#11495,#9575,#9576);
#8933=AXIS2_PLACEMENT_3D('',#11501,#9580,#9581);
#8934=AXIS2_PLACEMENT_3D('',#11510,#9586,#9587);
#8935=AXIS2_PLACEMENT_3D('',#11516,#9591,#9592);
#8936=AXIS2_PLACEMENT_3D('',#11525,#9597,#9598);
#8937=AXIS2_PLACEMENT_3D('',#11531,#9602,#9603);
#8938=AXIS2_PLACEMENT_3D('',#11540,#9608,#9609);
#8939=AXIS2_PLACEMENT_3D('',#11546,#9613,#9614);
#8940=AXIS2_PLACEMENT_3D('',#11555,#9619,#9620);
#8941=AXIS2_PLACEMENT_3D('',#11561,#9624,#9625);
#8942=AXIS2_PLACEMENT_3D('',#11570,#9630,#9631);
#8943=AXIS2_PLACEMENT_3D('',#11576,#9635,#9636);
#8944=AXIS2_PLACEMENT_3D('',#11585,#9641,#9642);
#8945=AXIS2_PLACEMENT_3D('',#11591,#9646,#9647);
#8946=AXIS2_PLACEMENT_3D('',#11600,#9652,#9653);
#8947=AXIS2_PLACEMENT_3D('',#11606,#9657,#9658);
#8948=AXIS2_PLACEMENT_3D('',#11615,#9663,#9664);
#8949=AXIS2_PLACEMENT_3D('',#11621,#9668,#9669);
#8950=AXIS2_PLACEMENT_3D('',#11630,#9674,#9675);
#8951=AXIS2_PLACEMENT_3D('',#11636,#9679,#9680);
#8952=AXIS2_PLACEMENT_3D('',#11645,#9685,#9686);
#8953=AXIS2_PLACEMENT_3D('',#11651,#9690,#9691);
#8954=AXIS2_PLACEMENT_3D('',#11660,#9696,#9697);
#8955=AXIS2_PLACEMENT_3D('',#11666,#9701,#9702);
#8956=AXIS2_PLACEMENT_3D('',#11675,#9707,#9708);
#8957=AXIS2_PLACEMENT_3D('',#11681,#9712,#9713);
#8958=AXIS2_PLACEMENT_3D('',#11690,#9718,#9719);
#8959=AXIS2_PLACEMENT_3D('',#11696,#9723,#9724);
#8960=AXIS2_PLACEMENT_3D('',#11705,#9729,#9730);
#8961=AXIS2_PLACEMENT_3D('',#11711,#9734,#9735);
#8962=AXIS2_PLACEMENT_3D('',#11720,#9740,#9741);
#8963=AXIS2_PLACEMENT_3D('',#11726,#9745,#9746);
#8964=AXIS2_PLACEMENT_3D('',#11735,#9751,#9752);
#8965=AXIS2_PLACEMENT_3D('',#11741,#9756,#9757);
#8966=AXIS2_PLACEMENT_3D('',#11750,#9762,#9763);
#8967=AXIS2_PLACEMENT_3D('',#11756,#9767,#9768);
#8968=AXIS2_PLACEMENT_3D('',#11765,#9773,#9774);
#8969=AXIS2_PLACEMENT_3D('',#11771,#9778,#9779);
#8970=AXIS2_PLACEMENT_3D('',#11780,#9784,#9785);
#8971=AXIS2_PLACEMENT_3D('',#11786,#9789,#9790);
#8972=AXIS2_PLACEMENT_3D('',#11795,#9795,#9796);
#8973=AXIS2_PLACEMENT_3D('',#11801,#9800,#9801);
#8974=AXIS2_PLACEMENT_3D('',#11810,#9806,#9807);
#8975=AXIS2_PLACEMENT_3D('',#11816,#9811,#9812);
#8976=AXIS2_PLACEMENT_3D('',#11825,#9817,#9818);
#8977=AXIS2_PLACEMENT_3D('',#11831,#9822,#9823);
#8978=AXIS2_PLACEMENT_3D('',#11840,#9828,#9829);
#8979=AXIS2_PLACEMENT_3D('',#11846,#9833,#9834);
#8980=AXIS2_PLACEMENT_3D('',#11855,#9839,#9840);
#8981=AXIS2_PLACEMENT_3D('',#11861,#9844,#9845);
#8982=AXIS2_PLACEMENT_3D('',#11870,#9850,#9851);
#8983=AXIS2_PLACEMENT_3D('',#11876,#9855,#9856);
#8984=AXIS2_PLACEMENT_3D('',#11885,#9861,#9862);
#8985=AXIS2_PLACEMENT_3D('',#11891,#9866,#9867);
#8986=AXIS2_PLACEMENT_3D('',#11900,#9872,#9873);
#8987=AXIS2_PLACEMENT_3D('',#11906,#9877,#9878);
#8988=AXIS2_PLACEMENT_3D('',#11915,#9883,#9884);
#8989=AXIS2_PLACEMENT_3D('',#11921,#9888,#9889);
#8990=AXIS2_PLACEMENT_3D('',#11930,#9894,#9895);
#8991=AXIS2_PLACEMENT_3D('',#11936,#9899,#9900);
#8992=AXIS2_PLACEMENT_3D('',#11945,#9905,#9906);
#8993=AXIS2_PLACEMENT_3D('',#11951,#9910,#9911);
#8994=AXIS2_PLACEMENT_3D('',#11960,#9916,#9917);
#8995=AXIS2_PLACEMENT_3D('',#11966,#9921,#9922);
#8996=AXIS2_PLACEMENT_3D('',#11975,#9927,#9928);
#8997=AXIS2_PLACEMENT_3D('',#11981,#9932,#9933);
#8998=AXIS2_PLACEMENT_3D('',#11990,#9938,#9939);
#8999=AXIS2_PLACEMENT_3D('',#11996,#9943,#9944);
#9000=AXIS2_PLACEMENT_3D('',#12006,#9950,#9951);
#9001=AXIS2_PLACEMENT_3D('',#12009,#9954,#9955);
#9002=AXIS2_PLACEMENT_3D('',#12012,#9958,#9959);
#9003=AXIS2_PLACEMENT_3D('',#12015,#9962,#9963);
#9004=AXIS2_PLACEMENT_3D('',#12018,#9966,#9967);
#9005=AXIS2_PLACEMENT_3D('',#12021,#9970,#9971);
#9006=AXIS2_PLACEMENT_3D('',#12024,#9974,#9975);
#9007=AXIS2_PLACEMENT_3D('',#12027,#9978,#9979);
#9008=AXIS2_PLACEMENT_3D('',#12030,#9982,#9983);
#9009=AXIS2_PLACEMENT_3D('',#12033,#9986,#9987);
#9010=AXIS2_PLACEMENT_3D('',#12036,#9990,#9991);
#9011=AXIS2_PLACEMENT_3D('',#12039,#9994,#9995);
#9012=AXIS2_PLACEMENT_3D('',#12042,#9998,#9999);
#9013=AXIS2_PLACEMENT_3D('',#12045,#10002,#10003);
#9014=AXIS2_PLACEMENT_3D('',#12048,#10006,#10007);
#9015=AXIS2_PLACEMENT_3D('',#12051,#10010,#10011);
#9016=AXIS2_PLACEMENT_3D('',#12054,#10014,#10015);
#9017=AXIS2_PLACEMENT_3D('',#12057,#10018,#10019);
#9018=AXIS2_PLACEMENT_3D('',#12060,#10022,#10023);
#9019=AXIS2_PLACEMENT_3D('',#12063,#10026,#10027);
#9020=AXIS2_PLACEMENT_3D('',#12066,#10030,#10031);
#9021=AXIS2_PLACEMENT_3D('',#12069,#10034,#10035);
#9022=AXIS2_PLACEMENT_3D('',#12072,#10038,#10039);
#9023=AXIS2_PLACEMENT_3D('',#12075,#10042,#10043);
#9024=AXIS2_PLACEMENT_3D('',#12078,#10046,#10047);
#9025=AXIS2_PLACEMENT_3D('',#12081,#10050,#10051);
#9026=AXIS2_PLACEMENT_3D('',#12084,#10054,#10055);
#9027=AXIS2_PLACEMENT_3D('',#12087,#10058,#10059);
#9028=AXIS2_PLACEMENT_3D('',#12090,#10062,#10063);
#9029=AXIS2_PLACEMENT_3D('',#12096,#10067,#10068);
#9030=AXIS2_PLACEMENT_3D('',#12099,#10071,#10072);
#9031=AXIS2_PLACEMENT_3D('',#12102,#10075,#10076);
#9032=AXIS2_PLACEMENT_3D('',#12105,#10079,#10080);
#9033=AXIS2_PLACEMENT_3D('',#12108,#10083,#10084);
#9034=AXIS2_PLACEMENT_3D('',#12111,#10087,#10088);
#9035=AXIS2_PLACEMENT_3D('',#12114,#10091,#10092);
#9036=AXIS2_PLACEMENT_3D('',#12117,#10095,#10096);
#9037=AXIS2_PLACEMENT_3D('',#12120,#10099,#10100);
#9038=AXIS2_PLACEMENT_3D('',#12123,#10103,#10104);
#9039=AXIS2_PLACEMENT_3D('',#12131,#10109,#10110);
#9040=AXIS2_PLACEMENT_3D('',#12135,#10113,#10114);
#9041=AXIS2_PLACEMENT_3D('',#12144,#10119,#10120);
#9042=AXIS2_PLACEMENT_3D('',#12148,#10123,#10124);
#9043=AXIS2_PLACEMENT_3D('',#12152,#10127,#10128);
#9044=AXIS2_PLACEMENT_3D('',#12155,#10131,#10132);
#9045=AXIS2_PLACEMENT_3D('',#12157,#10133,#10134);
#9046=AXIS2_PLACEMENT_3D('',#12170,#10141,#10142);
#9047=AXIS2_PLACEMENT_3D('',#12171,#10143,#10144);
#9048=AXIS2_PLACEMENT_3D('',#12173,#10145,#10146);
#9049=AXIS2_PLACEMENT_3D('',#12175,#10148,#10149);
#9050=AXIS2_PLACEMENT_3D('',#12181,#10153,#10154);
#9051=AXIS2_PLACEMENT_3D('',#12185,#10157,#10158);
#9052=AXIS2_PLACEMENT_3D('',#12189,#10161,#10162);
#9053=AXIS2_PLACEMENT_3D('',#12193,#10165,#10166);
#9054=AXIS2_PLACEMENT_3D('',#12197,#10169,#10170);
#9055=AXIS2_PLACEMENT_3D('',#12199,#10172,#10173);
#9056=AXIS2_PLACEMENT_3D('',#12200,#10174,#10175);
#9057=AXIS2_PLACEMENT_3D('',#12201,#10176,#10177);
#9502=DIRECTION('axis',(0.,0.,1.));
#9503=DIRECTION('refdir',(1.,0.,0.));
#9504=DIRECTION('center_axis',(0.,0.,-1.));
#9505=DIRECTION('ref_axis',(1.,0.,0.));
#9506=DIRECTION('center_axis',(0.,0.,-1.));
#9507=DIRECTION('ref_axis',(1.,0.,0.));
#9508=DIRECTION('',(0.,0.,-1.));
#9509=DIRECTION('center_axis',(0.,0.,1.));
#9510=DIRECTION('ref_axis',(1.,0.,0.));
#9511=DIRECTION('center_axis',(0.,0.,-1.));
#9512=DIRECTION('ref_axis',(1.,0.,0.));
#9513=DIRECTION('center_axis',(0.,0.,-1.));
#9514=DIRECTION('ref_axis',(1.,0.,0.));
#9515=DIRECTION('',(0.,0.,-1.));
#9516=DIRECTION('center_axis',(0.,0.,1.));
#9517=DIRECTION('ref_axis',(1.,0.,0.));
#9518=DIRECTION('center_axis',(0.,0.,-1.));
#9519=DIRECTION('ref_axis',(1.,0.,0.));
#9520=DIRECTION('center_axis',(0.,0.,-1.));
#9521=DIRECTION('ref_axis',(1.,0.,0.));
#9522=DIRECTION('',(0.,0.,-1.));
#9523=DIRECTION('center_axis',(0.,0.,1.));
#9524=DIRECTION('ref_axis',(1.,0.,0.));
#9525=DIRECTION('center_axis',(0.810679228399881,0.585490553844358,0.));
#9526=DIRECTION('ref_axis',(0.585490553844358,-0.810679228399881,0.));
#9527=DIRECTION('',(0.,0.,-1.));
#9528=DIRECTION('',(0.585490553844358,-0.810679228399881,0.));
#9529=DIRECTION('',(0.,0.,-1.));
#9530=DIRECTION('',(-0.585490553844358,0.810679228399881,0.));
#9531=DIRECTION('center_axis',(-0.810679228399881,0.585490553844358,0.));
#9532=DIRECTION('ref_axis',(0.585490553844358,0.810679228399881,0.));
#9533=DIRECTION('',(0.,0.,1.));
#9534=DIRECTION('',(-0.585490553844358,-0.810679228399881,0.));
#9535=DIRECTION('',(0.585490553844358,0.810679228399881,0.));
#9536=DIRECTION('center_axis',(0.810679228399881,0.585490553844358,0.));
#9537=DIRECTION('ref_axis',(0.585490553844358,-0.810679228399881,0.));
#9538=DIRECTION('',(0.,0.,-1.));
#9539=DIRECTION('',(0.585490553844358,-0.810679228399881,0.));
#9540=DIRECTION('',(0.,0.,-1.));
#9541=DIRECTION('',(-0.585490553844358,0.810679228399881,0.));
#9542=DIRECTION('center_axis',(-0.810679228399881,0.585490553844358,0.));
#9543=DIRECTION('ref_axis',(0.585490553844358,0.810679228399881,0.));
#9544=DIRECTION('',(0.,0.,1.));
#9545=DIRECTION('',(-0.585490553844358,-0.810679228399881,0.));
#9546=DIRECTION('',(0.585490553844358,0.810679228399881,0.));
#9547=DIRECTION('center_axis',(0.810679228399883,0.585490553844356,0.));
#9548=DIRECTION('ref_axis',(0.585490553844356,-0.810679228399883,0.));
#9549=DIRECTION('',(0.,0.,-1.));
#9550=DIRECTION('',(0.585490553844356,-0.810679228399883,0.));
#9551=DIRECTION('',(0.,0.,-1.));
#9552=DIRECTION('',(-0.585490553844356,0.810679228399883,0.));
#9553=DIRECTION('center_axis',(-0.810679228399881,0.585490553844358,0.));
#9554=DIRECTION('ref_axis',(0.585490553844358,0.810679228399881,0.));
#9555=DIRECTION('',(0.,0.,1.));
#9556=DIRECTION('',(-0.585490553844358,-0.810679228399881,0.));
#9557=DIRECTION('',(0.585490553844358,0.810679228399881,0.));
#9558=DIRECTION('center_axis',(0.810679228399879,0.585490553844361,0.));
#9559=DIRECTION('ref_axis',(0.585490553844361,-0.810679228399879,0.));
#9560=DIRECTION('',(0.,0.,-1.));
#9561=DIRECTION('',(0.585490553844361,-0.810679228399879,0.));
#9562=DIRECTION('',(0.,0.,-1.));
#9563=DIRECTION('',(-0.585490553844361,0.810679228399879,0.));
#9564=DIRECTION('center_axis',(-0.810679228399883,0.585490553844356,0.));
#9565=DIRECTION('ref_axis',(0.585490553844356,0.810679228399883,0.));
#9566=DIRECTION('',(0.,0.,1.));
#9567=DIRECTION('',(-0.585490553844356,-0.810679228399883,0.));
#9568=DIRECTION('',(0.585490553844356,0.810679228399883,0.));
#9569=DIRECTION('center_axis',(0.810679228399883,0.585490553844356,0.));
#9570=DIRECTION('ref_axis',(0.585490553844356,-0.810679228399883,0.));
#9571=DIRECTION('',(0.,0.,-1.));
#9572=DIRECTION('',(0.585490553844356,-0.810679228399883,0.));
#9573=DIRECTION('',(0.,0.,-1.));
#9574=DIRECTION('',(-0.585490553844356,0.810679228399883,0.));
#9575=DIRECTION('center_axis',(-0.810679228399879,0.585490553844361,0.));
#9576=DIRECTION('ref_axis',(0.585490553844361,0.810679228399879,0.));
#9577=DIRECTION('',(0.,0.,1.));
#9578=DIRECTION('',(-0.585490553844361,-0.810679228399879,0.));
#9579=DIRECTION('',(0.585490553844361,0.810679228399879,0.));
#9580=DIRECTION('center_axis',(0.810679228399883,0.585490553844356,0.));
#9581=DIRECTION('ref_axis',(0.585490553844356,-0.810679228399883,0.));
#9582=DIRECTION('',(0.,0.,-1.));
#9583=DIRECTION('',(0.585490553844356,-0.810679228399883,0.));
#9584=DIRECTION('',(0.,0.,-1.));
#9585=DIRECTION('',(-0.585490553844356,0.810679228399883,0.));
#9586=DIRECTION('center_axis',(-0.810679228399883,0.585490553844356,0.));
#9587=DIRECTION('ref_axis',(0.585490553844356,0.810679228399883,0.));
#9588=DIRECTION('',(0.,0.,1.));
#9589=DIRECTION('',(-0.585490553844356,-0.810679228399883,0.));
#9590=DIRECTION('',(0.585490553844356,0.810679228399883,0.));
#9591=DIRECTION('center_axis',(0.810679228399879,0.585490553844361,0.));
#9592=DIRECTION('ref_axis',(0.585490553844361,-0.810679228399879,0.));
#9593=DIRECTION('',(0.,0.,-1.));
#9594=DIRECTION('',(0.585490553844361,-0.810679228399879,0.));
#9595=DIRECTION('',(0.,0.,-1.));
#9596=DIRECTION('',(-0.585490553844361,0.810679228399879,0.));
#9597=DIRECTION('center_axis',(-0.810679228399883,0.585490553844356,0.));
#9598=DIRECTION('ref_axis',(0.585490553844356,0.810679228399883,0.));
#9599=DIRECTION('',(0.,0.,1.));
#9600=DIRECTION('',(-0.585490553844356,-0.810679228399883,0.));
#9601=DIRECTION('',(0.585490553844356,0.810679228399883,0.));
#9602=DIRECTION('center_axis',(0.810679228399883,0.585490553844356,0.));
#9603=DIRECTION('ref_axis',(0.585490553844356,-0.810679228399883,0.));
#9604=DIRECTION('',(0.,0.,-1.));
#9605=DIRECTION('',(0.585490553844356,-0.810679228399883,0.));
#9606=DIRECTION('',(0.,0.,-1.));
#9607=DIRECTION('',(-0.585490553844356,0.810679228399883,0.));
#9608=DIRECTION('center_axis',(-0.810679228399879,0.585490553844361,0.));
#9609=DIRECTION('ref_axis',(0.585490553844361,0.810679228399879,0.));
#9610=DIRECTION('',(0.,0.,1.));
#9611=DIRECTION('',(-0.585490553844361,-0.810679228399879,0.));
#9612=DIRECTION('',(0.585490553844361,0.810679228399879,0.));
#9613=DIRECTION('center_axis',(0.810679228399879,0.585490553844361,0.));
#9614=DIRECTION('ref_axis',(0.585490553844361,-0.810679228399879,0.));
#9615=DIRECTION('',(0.,0.,-1.));
#9616=DIRECTION('',(0.585490553844361,-0.810679228399879,0.));
#9617=DIRECTION('',(0.,0.,-1.));
#9618=DIRECTION('',(-0.585490553844361,0.810679228399879,0.));
#9619=DIRECTION('center_axis',(-0.810679228399883,0.585490553844356,0.));
#9620=DIRECTION('ref_axis',(0.585490553844356,0.810679228399883,0.));
#9621=DIRECTION('',(0.,0.,1.));
#9622=DIRECTION('',(-0.585490553844356,-0.810679228399883,0.));
#9623=DIRECTION('',(0.585490553844356,0.810679228399883,0.));
#9624=DIRECTION('center_axis',(0.810679228399883,0.585490553844356,0.));
#9625=DIRECTION('ref_axis',(0.585490553844356,-0.810679228399883,0.));
#9626=DIRECTION('',(0.,0.,-1.));
#9627=DIRECTION('',(0.585490553844356,-0.810679228399883,0.));
#9628=DIRECTION('',(0.,0.,-1.));
#9629=DIRECTION('',(-0.585490553844356,0.810679228399883,0.));
#9630=DIRECTION('center_axis',(-0.810679228399875,0.585490553844366,0.));
#9631=DIRECTION('ref_axis',(0.585490553844366,0.810679228399875,0.));
#9632=DIRECTION('',(0.,0.,1.));
#9633=DIRECTION('',(-0.585490553844366,-0.810679228399875,0.));
#9634=DIRECTION('',(0.585490553844366,0.810679228399875,0.));
#9635=DIRECTION('center_axis',(0.810679228399879,0.585490553844361,0.));
#9636=DIRECTION('ref_axis',(0.585490553844361,-0.810679228399879,0.));
#9637=DIRECTION('',(0.,0.,-1.));
#9638=DIRECTION('',(0.585490553844361,-0.810679228399879,0.));
#9639=DIRECTION('',(0.,0.,-1.));
#9640=DIRECTION('',(-0.585490553844361,0.810679228399879,0.));
#9641=DIRECTION('center_axis',(-0.810679228399879,0.585490553844361,0.));
#9642=DIRECTION('ref_axis',(0.585490553844361,0.810679228399879,0.));
#9643=DIRECTION('',(0.,0.,1.));
#9644=DIRECTION('',(-0.585490553844361,-0.810679228399879,0.));
#9645=DIRECTION('',(0.585490553844361,0.810679228399879,0.));
#9646=DIRECTION('center_axis',(0.810679228399879,0.585490553844361,0.));
#9647=DIRECTION('ref_axis',(0.585490553844361,-0.810679228399879,0.));
#9648=DIRECTION('',(0.,0.,-1.));
#9649=DIRECTION('',(0.585490553844361,-0.810679228399879,0.));
#9650=DIRECTION('',(0.,0.,-1.));
#9651=DIRECTION('',(-0.585490553844361,0.810679228399879,0.));
#9652=DIRECTION('center_axis',(-0.810679228399879,0.585490553844361,0.));
#9653=DIRECTION('ref_axis',(0.585490553844361,0.810679228399879,0.));
#9654=DIRECTION('',(0.,0.,1.));
#9655=DIRECTION('',(-0.585490553844361,-0.810679228399879,0.));
#9656=DIRECTION('',(0.585490553844361,0.810679228399879,0.));
#9657=DIRECTION('center_axis',(0.810679228399879,0.585490553844361,0.));
#9658=DIRECTION('ref_axis',(0.585490553844361,-0.810679228399879,0.));
#9659=DIRECTION('',(0.,0.,-1.));
#9660=DIRECTION('',(0.585490553844361,-0.810679228399879,0.));
#9661=DIRECTION('',(0.,0.,-1.));
#9662=DIRECTION('',(-0.585490553844361,0.810679228399879,0.));
#9663=DIRECTION('center_axis',(-0.810679228399875,0.585490553844366,0.));
#9664=DIRECTION('ref_axis',(0.585490553844366,0.810679228399875,0.));
#9665=DIRECTION('',(0.,0.,1.));
#9666=DIRECTION('',(-0.585490553844366,-0.810679228399875,0.));
#9667=DIRECTION('',(0.585490553844366,0.810679228399875,0.));
#9668=DIRECTION('center_axis',(0.810679228399879,0.585490553844361,0.));
#9669=DIRECTION('ref_axis',(0.585490553844361,-0.810679228399879,0.));
#9670=DIRECTION('',(0.,0.,-1.));
#9671=DIRECTION('',(0.585490553844361,-0.810679228399879,0.));
#9672=DIRECTION('',(0.,0.,-1.));
#9673=DIRECTION('',(-0.585490553844361,0.810679228399879,0.));
#9674=DIRECTION('center_axis',(-0.810679228399875,0.585490553844366,0.));
#9675=DIRECTION('ref_axis',(0.585490553844366,0.810679228399875,0.));
#9676=DIRECTION('',(0.,0.,1.));
#9677=DIRECTION('',(-0.585490553844366,-0.810679228399875,0.));
#9678=DIRECTION('',(0.585490553844366,0.810679228399875,0.));
#9679=DIRECTION('center_axis',(0.810679228399875,0.585490553844366,0.));
#9680=DIRECTION('ref_axis',(0.585490553844366,-0.810679228399875,0.));
#9681=DIRECTION('',(0.,0.,-1.));
#9682=DIRECTION('',(0.585490553844366,-0.810679228399875,0.));
#9683=DIRECTION('',(0.,0.,-1.));
#9684=DIRECTION('',(-0.585490553844366,0.810679228399875,0.));
#9685=DIRECTION('center_axis',(-0.810679228399883,0.585490553844356,0.));
#9686=DIRECTION('ref_axis',(0.585490553844356,0.810679228399883,0.));
#9687=DIRECTION('',(0.,0.,1.));
#9688=DIRECTION('',(-0.585490553844356,-0.810679228399883,0.));
#9689=DIRECTION('',(0.585490553844356,0.810679228399883,0.));
#9690=DIRECTION('center_axis',(0.810679228399875,0.585490553844366,0.));
#9691=DIRECTION('ref_axis',(0.585490553844366,-0.810679228399875,0.));
#9692=DIRECTION('',(0.,0.,-1.));
#9693=DIRECTION('',(0.585490553844366,-0.810679228399875,0.));
#9694=DIRECTION('',(0.,0.,-1.));
#9695=DIRECTION('',(-0.585490553844366,0.810679228399875,0.));
#9696=DIRECTION('center_axis',(-0.810679228399883,0.585490553844356,0.));
#9697=DIRECTION('ref_axis',(0.585490553844356,0.810679228399883,0.));
#9698=DIRECTION('',(0.,0.,1.));
#9699=DIRECTION('',(-0.585490553844356,-0.810679228399883,0.));
#9700=DIRECTION('',(0.585490553844356,0.810679228399883,0.));
#9701=DIRECTION('center_axis',(0.810679228399883,0.585490553844356,0.));
#9702=DIRECTION('ref_axis',(0.585490553844356,-0.810679228399883,0.));
#9703=DIRECTION('',(0.,0.,-1.));
#9704=DIRECTION('',(0.585490553844356,-0.810679228399883,0.));
#9705=DIRECTION('',(0.,0.,-1.));
#9706=DIRECTION('',(-0.585490553844356,0.810679228399883,0.));
#9707=DIRECTION('center_axis',(-0.810679228399875,0.585490553844366,0.));
#9708=DIRECTION('ref_axis',(0.585490553844366,0.810679228399875,0.));
#9709=DIRECTION('',(0.,0.,1.));
#9710=DIRECTION('',(-0.585490553844366,-0.810679228399875,0.));
#9711=DIRECTION('',(0.585490553844366,0.810679228399875,0.));
#9712=DIRECTION('center_axis',(0.810679228399883,0.585490553844356,0.));
#9713=DIRECTION('ref_axis',(0.585490553844356,-0.810679228399883,0.));
#9714=DIRECTION('',(0.,0.,-1.));
#9715=DIRECTION('',(0.585490553844356,-0.810679228399883,0.));
#9716=DIRECTION('',(0.,0.,-1.));
#9717=DIRECTION('',(-0.585490553844356,0.810679228399883,0.));
#9718=DIRECTION('center_axis',(-0.810679228399875,0.585490553844366,0.));
#9719=DIRECTION('ref_axis',(0.585490553844366,0.810679228399875,0.));
#9720=DIRECTION('',(0.,0.,1.));
#9721=DIRECTION('',(-0.585490553844366,-0.810679228399875,0.));
#9722=DIRECTION('',(0.585490553844366,0.810679228399875,0.));
#9723=DIRECTION('center_axis',(0.810679228399875,0.585490553844366,0.));
#9724=DIRECTION('ref_axis',(0.585490553844366,-0.810679228399875,0.));
#9725=DIRECTION('',(0.,0.,-1.));
#9726=DIRECTION('',(0.585490553844366,-0.810679228399875,0.));
#9727=DIRECTION('',(0.,0.,-1.));
#9728=DIRECTION('',(-0.585490553844366,0.810679228399875,0.));
#9729=DIRECTION('center_axis',(-0.810679228399875,0.585490553844366,0.));
#9730=DIRECTION('ref_axis',(0.585490553844366,0.810679228399875,0.));
#9731=DIRECTION('',(0.,0.,1.));
#9732=DIRECTION('',(-0.585490553844366,-0.810679228399875,0.));
#9733=DIRECTION('',(0.585490553844366,0.810679228399875,0.));
#9734=DIRECTION('center_axis',(0.810679228399875,0.585490553844366,0.));
#9735=DIRECTION('ref_axis',(0.585490553844366,-0.810679228399875,0.));
#9736=DIRECTION('',(0.,0.,-1.));
#9737=DIRECTION('',(0.585490553844366,-0.810679228399875,0.));
#9738=DIRECTION('',(0.,0.,-1.));
#9739=DIRECTION('',(-0.585490553844366,0.810679228399875,0.));
#9740=DIRECTION('center_axis',(-0.810679228399883,0.585490553844356,0.));
#9741=DIRECTION('ref_axis',(0.585490553844356,0.810679228399883,0.));
#9742=DIRECTION('',(0.,0.,1.));
#9743=DIRECTION('',(-0.585490553844356,-0.810679228399883,0.));
#9744=DIRECTION('',(0.585490553844356,0.810679228399883,0.));
#9745=DIRECTION('center_axis',(0.810679228399875,0.585490553844366,0.));
#9746=DIRECTION('ref_axis',(0.585490553844366,-0.810679228399875,0.));
#9747=DIRECTION('',(0.,0.,-1.));
#9748=DIRECTION('',(0.585490553844366,-0.810679228399875,0.));
#9749=DIRECTION('',(0.,0.,-1.));
#9750=DIRECTION('',(-0.585490553844366,0.810679228399875,0.));
#9751=DIRECTION('center_axis',(-0.810679228399883,0.585490553844356,0.));
#9752=DIRECTION('ref_axis',(0.585490553844356,0.810679228399883,0.));
#9753=DIRECTION('',(0.,0.,1.));
#9754=DIRECTION('',(-0.585490553844356,-0.810679228399883,0.));
#9755=DIRECTION('',(0.585490553844356,0.810679228399883,0.));
#9756=DIRECTION('center_axis',(0.810679228399875,0.585490553844366,0.));
#9757=DIRECTION('ref_axis',(0.585490553844366,-0.810679228399875,0.));
#9758=DIRECTION('',(0.,0.,-1.));
#9759=DIRECTION('',(0.585490553844366,-0.810679228399875,0.));
#9760=DIRECTION('',(0.,0.,-1.));
#9761=DIRECTION('',(-0.585490553844366,0.810679228399875,0.));
#9762=DIRECTION('center_axis',(-0.810679228399875,0.585490553844366,0.));
#9763=DIRECTION('ref_axis',(0.585490553844366,0.810679228399875,0.));
#9764=DIRECTION('',(0.,0.,1.));
#9765=DIRECTION('',(-0.585490553844366,-0.810679228399875,0.));
#9766=DIRECTION('',(0.585490553844366,0.810679228399875,0.));
#9767=DIRECTION('center_axis',(0.810679228399883,0.585490553844356,0.));
#9768=DIRECTION('ref_axis',(0.585490553844356,-0.810679228399883,0.));
#9769=DIRECTION('',(0.,0.,-1.));
#9770=DIRECTION('',(0.585490553844356,-0.810679228399883,0.));
#9771=DIRECTION('',(0.,0.,-1.));
#9772=DIRECTION('',(-0.585490553844356,0.810679228399883,0.));
#9773=DIRECTION('center_axis',(-0.810679228399875,0.585490553844366,0.));
#9774=DIRECTION('ref_axis',(0.585490553844366,0.810679228399875,0.));
#9775=DIRECTION('',(0.,0.,1.));
#9776=DIRECTION('',(-0.585490553844366,-0.810679228399875,0.));
#9777=DIRECTION('',(0.585490553844366,0.810679228399875,0.));
#9778=DIRECTION('center_axis',(0.810679228399883,0.585490553844356,0.));
#9779=DIRECTION('ref_axis',(0.585490553844356,-0.810679228399883,0.));
#9780=DIRECTION('',(0.,0.,-1.));
#9781=DIRECTION('',(0.585490553844356,-0.810679228399883,0.));
#9782=DIRECTION('',(0.,0.,-1.));
#9783=DIRECTION('',(-0.585490553844356,0.810679228399883,0.));
#9784=DIRECTION('center_axis',(-0.810679228399875,0.585490553844366,0.));
#9785=DIRECTION('ref_axis',(0.585490553844366,0.810679228399875,0.));
#9786=DIRECTION('',(0.,0.,1.));
#9787=DIRECTION('',(-0.585490553844366,-0.810679228399875,0.));
#9788=DIRECTION('',(0.585490553844366,0.810679228399875,0.));
#9789=DIRECTION('center_axis',(0.810679228399879,0.585490553844361,0.));
#9790=DIRECTION('ref_axis',(0.585490553844361,-0.810679228399879,0.));
#9791=DIRECTION('',(0.,0.,-1.));
#9792=DIRECTION('',(0.585490553844361,-0.810679228399879,0.));
#9793=DIRECTION('',(0.,0.,-1.));
#9794=DIRECTION('',(-0.585490553844361,0.810679228399879,0.));
#9795=DIRECTION('center_axis',(-0.810679228399879,0.585490553844361,0.));
#9796=DIRECTION('ref_axis',(0.585490553844361,0.810679228399879,0.));
#9797=DIRECTION('',(0.,0.,1.));
#9798=DIRECTION('',(-0.585490553844361,-0.810679228399879,0.));
#9799=DIRECTION('',(0.585490553844361,0.810679228399879,0.));
#9800=DIRECTION('center_axis',(0.810679228399875,0.585490553844366,0.));
#9801=DIRECTION('ref_axis',(0.585490553844366,-0.810679228399875,0.));
#9802=DIRECTION('',(0.,0.,-1.));
#9803=DIRECTION('',(0.585490553844366,-0.810679228399875,0.));
#9804=DIRECTION('',(0.,0.,-1.));
#9805=DIRECTION('',(-0.585490553844366,0.810679228399875,0.));
#9806=DIRECTION('center_axis',(-0.810679228399879,0.585490553844361,0.));
#9807=DIRECTION('ref_axis',(0.585490553844361,0.810679228399879,0.));
#9808=DIRECTION('',(0.,0.,1.));
#9809=DIRECTION('',(-0.585490553844361,-0.810679228399879,0.));
#9810=DIRECTION('',(0.585490553844361,0.810679228399879,0.));
#9811=DIRECTION('center_axis',(0.810679228399879,0.585490553844361,0.));
#9812=DIRECTION('ref_axis',(0.585490553844361,-0.810679228399879,0.));
#9813=DIRECTION('',(0.,0.,-1.));
#9814=DIRECTION('',(0.585490553844361,-0.810679228399879,0.));
#9815=DIRECTION('',(0.,0.,-1.));
#9816=DIRECTION('',(-0.585490553844361,0.810679228399879,0.));
#9817=DIRECTION('center_axis',(-0.810679228399879,0.585490553844361,0.));
#9818=DIRECTION('ref_axis',(0.585490553844361,0.810679228399879,0.));
#9819=DIRECTION('',(0.,0.,1.));
#9820=DIRECTION('',(-0.585490553844361,-0.810679228399879,0.));
#9821=DIRECTION('',(0.585490553844361,0.810679228399879,0.));
#9822=DIRECTION('center_axis',(0.810679228399879,0.585490553844361,0.));
#9823=DIRECTION('ref_axis',(0.585490553844361,-0.810679228399879,0.));
#9824=DIRECTION('',(0.,0.,-1.));
#9825=DIRECTION('',(0.585490553844361,-0.810679228399879,0.));
#9826=DIRECTION('',(0.,0.,-1.));
#9827=DIRECTION('',(-0.585490553844361,0.810679228399879,0.));
#9828=DIRECTION('center_axis',(-0.810679228399875,0.585490553844366,0.));
#9829=DIRECTION('ref_axis',(0.585490553844366,0.810679228399875,0.));
#9830=DIRECTION('',(0.,0.,1.));
#9831=DIRECTION('',(-0.585490553844366,-0.810679228399875,0.));
#9832=DIRECTION('',(0.585490553844366,0.810679228399875,0.));
#9833=DIRECTION('center_axis',(0.810679228399879,0.585490553844361,0.));
#9834=DIRECTION('ref_axis',(0.585490553844361,-0.810679228399879,0.));
#9835=DIRECTION('',(0.,0.,-1.));
#9836=DIRECTION('',(0.585490553844361,-0.810679228399879,0.));
#9837=DIRECTION('',(0.,0.,-1.));
#9838=DIRECTION('',(-0.585490553844361,0.810679228399879,0.));
#9839=DIRECTION('center_axis',(-0.810679228399879,0.585490553844361,0.));
#9840=DIRECTION('ref_axis',(0.585490553844361,0.810679228399879,0.));
#9841=DIRECTION('',(0.,0.,1.));
#9842=DIRECTION('',(-0.585490553844361,-0.810679228399879,0.));
#9843=DIRECTION('',(0.585490553844361,0.810679228399879,0.));
#9844=DIRECTION('center_axis',(0.810679228399883,0.585490553844356,0.));
#9845=DIRECTION('ref_axis',(0.585490553844356,-0.810679228399883,0.));
#9846=DIRECTION('',(0.,0.,-1.));
#9847=DIRECTION('',(0.585490553844356,-0.810679228399883,0.));
#9848=DIRECTION('',(0.,0.,-1.));
#9849=DIRECTION('',(-0.585490553844356,0.810679228399883,0.));
#9850=DIRECTION('center_axis',(-0.810679228399883,0.585490553844356,0.));
#9851=DIRECTION('ref_axis',(0.585490553844356,0.810679228399883,0.));
#9852=DIRECTION('',(0.,0.,1.));
#9853=DIRECTION('',(-0.585490553844356,-0.810679228399883,0.));
#9854=DIRECTION('',(0.585490553844356,0.810679228399883,0.));
#9855=DIRECTION('center_axis',(0.810679228399883,0.585490553844356,0.));
#9856=DIRECTION('ref_axis',(0.585490553844356,-0.810679228399883,0.));
#9857=DIRECTION('',(0.,0.,-1.));
#9858=DIRECTION('',(0.585490553844356,-0.810679228399883,0.));
#9859=DIRECTION('',(0.,0.,-1.));
#9860=DIRECTION('',(-0.585490553844356,0.810679228399883,0.));
#9861=DIRECTION('center_axis',(-0.810679228399879,0.585490553844361,0.));
#9862=DIRECTION('ref_axis',(0.585490553844361,0.810679228399879,0.));
#9863=DIRECTION('',(0.,0.,1.));
#9864=DIRECTION('',(-0.585490553844361,-0.810679228399879,0.));
#9865=DIRECTION('',(0.585490553844361,0.810679228399879,0.));
#9866=DIRECTION('center_axis',(0.810679228399879,0.585490553844361,0.));
#9867=DIRECTION('ref_axis',(0.585490553844361,-0.810679228399879,0.));
#9868=DIRECTION('',(0.,0.,-1.));
#9869=DIRECTION('',(0.585490553844361,-0.810679228399879,0.));
#9870=DIRECTION('',(0.,0.,-1.));
#9871=DIRECTION('',(-0.585490553844361,0.810679228399879,0.));
#9872=DIRECTION('center_axis',(-0.810679228399883,0.585490553844356,0.));
#9873=DIRECTION('ref_axis',(0.585490553844356,0.810679228399883,0.));
#9874=DIRECTION('',(0.,0.,1.));
#9875=DIRECTION('',(-0.585490553844356,-0.810679228399883,0.));
#9876=DIRECTION('',(0.585490553844356,0.810679228399883,0.));
#9877=DIRECTION('center_axis',(0.810679228399883,0.585490553844356,0.));
#9878=DIRECTION('ref_axis',(0.585490553844356,-0.810679228399883,0.));
#9879=DIRECTION('',(0.,0.,-1.));
#9880=DIRECTION('',(0.585490553844356,-0.810679228399883,0.));
#9881=DIRECTION('',(0.,0.,-1.));
#9882=DIRECTION('',(-0.585490553844356,0.810679228399883,0.));
#9883=DIRECTION('center_axis',(-0.810679228399879,0.585490553844361,0.));
#9884=DIRECTION('ref_axis',(0.585490553844361,0.810679228399879,0.));
#9885=DIRECTION('',(0.,0.,1.));
#9886=DIRECTION('',(-0.585490553844361,-0.810679228399879,0.));
#9887=DIRECTION('',(0.585490553844361,0.810679228399879,0.));
#9888=DIRECTION('center_axis',(0.810679228399879,0.585490553844361,0.));
#9889=DIRECTION('ref_axis',(0.585490553844361,-0.810679228399879,0.));
#9890=DIRECTION('',(0.,0.,-1.));
#9891=DIRECTION('',(0.585490553844361,-0.810679228399879,0.));
#9892=DIRECTION('',(0.,0.,-1.));
#9893=DIRECTION('',(-0.585490553844361,0.810679228399879,0.));
#9894=DIRECTION('center_axis',(-0.810679228399883,0.585490553844356,0.));
#9895=DIRECTION('ref_axis',(0.585490553844356,0.810679228399883,0.));
#9896=DIRECTION('',(0.,0.,1.));
#9897=DIRECTION('',(-0.585490553844356,-0.810679228399883,0.));
#9898=DIRECTION('',(0.585490553844356,0.810679228399883,0.));
#9899=DIRECTION('center_axis',(0.810679228399881,0.585490553844358,0.));
#9900=DIRECTION('ref_axis',(0.585490553844358,-0.810679228399881,0.));
#9901=DIRECTION('',(0.,0.,-1.));
#9902=DIRECTION('',(0.585490553844358,-0.810679228399881,0.));
#9903=DIRECTION('',(0.,0.,-1.));
#9904=DIRECTION('',(-0.585490553844358,0.810679228399881,0.));
#9905=DIRECTION('center_axis',(-0.810679228399883,0.585490553844356,0.));
#9906=DIRECTION('ref_axis',(0.585490553844356,0.810679228399883,0.));
#9907=DIRECTION('',(0.,0.,1.));
#9908=DIRECTION('',(-0.585490553844356,-0.810679228399883,0.));
#9909=DIRECTION('',(0.585490553844356,0.810679228399883,0.));
#9910=DIRECTION('center_axis',(0.810679228399881,0.585490553844358,0.));
#9911=DIRECTION('ref_axis',(0.585490553844358,-0.810679228399881,0.));
#9912=DIRECTION('',(0.,0.,-1.));
#9913=DIRECTION('',(0.585490553844358,-0.810679228399881,0.));
#9914=DIRECTION('',(0.,0.,-1.));
#9915=DIRECTION('',(-0.585490553844358,0.810679228399881,0.));
#9916=DIRECTION('center_axis',(-0.810679228399881,0.585490553844358,0.));
#9917=DIRECTION('ref_axis',(0.585490553844358,0.810679228399881,0.));
#9918=DIRECTION('',(0.,0.,1.));
#9919=DIRECTION('',(-0.585490553844358,-0.810679228399881,0.));
#9920=DIRECTION('',(0.585490553844358,0.810679228399881,0.));
#9921=DIRECTION('center_axis',(0.810679228399881,0.585490553844358,0.));
#9922=DIRECTION('ref_axis',(0.585490553844358,-0.810679228399881,0.));
#9923=DIRECTION('',(0.,0.,-1.));
#9924=DIRECTION('',(0.585490553844358,-0.810679228399881,0.));
#9925=DIRECTION('',(0.,0.,-1.));
#9926=DIRECTION('',(-0.585490553844358,0.810679228399881,0.));
#9927=DIRECTION('center_axis',(-0.810679228399883,0.585490553844356,0.));
#9928=DIRECTION('ref_axis',(0.585490553844356,0.810679228399883,0.));
#9929=DIRECTION('',(0.,0.,1.));
#9930=DIRECTION('',(-0.585490553844356,-0.810679228399883,0.));
#9931=DIRECTION('',(0.585490553844356,0.810679228399883,0.));
#9932=DIRECTION('center_axis',(0.810679228399883,0.585490553844356,0.));
#9933=DIRECTION('ref_axis',(0.585490553844356,-0.810679228399883,0.));
#9934=DIRECTION('',(0.,0.,-1.));
#9935=DIRECTION('',(0.585490553844356,-0.810679228399883,0.));
#9936=DIRECTION('',(0.,0.,-1.));
#9937=DIRECTION('',(-0.585490553844356,0.810679228399883,0.));
#9938=DIRECTION('center_axis',(-0.810679228399881,0.585490553844358,0.));
#9939=DIRECTION('ref_axis',(0.585490553844358,0.810679228399881,0.));
#9940=DIRECTION('',(0.,0.,1.));
#9941=DIRECTION('',(-0.585490553844358,-0.810679228399881,0.));
#9942=DIRECTION('',(0.585490553844358,0.810679228399881,0.));
#9943=DIRECTION('center_axis',(0.,-1.,0.));
#9944=DIRECTION('ref_axis',(1.,0.,0.));
#9945=DIRECTION('',(-1.,0.,0.));
#9946=DIRECTION('',(0.,0.,1.));
#9947=DIRECTION('',(-1.,0.,0.));
#9948=DIRECTION('',(0.,0.,-1.));
#9949=DIRECTION('',(1.,0.,0.));
#9950=DIRECTION('center_axis',(0.,-1.,0.));
#9951=DIRECTION('ref_axis',(1.,0.,0.));
#9952=DIRECTION('',(-1.,0.,0.));
#9953=DIRECTION('',(1.,0.,0.));
#9954=DIRECTION('center_axis',(0.,-1.,0.));
#9955=DIRECTION('ref_axis',(1.,0.,0.));
#9956=DIRECTION('',(-1.,0.,0.));
#9957=DIRECTION('',(1.,0.,0.));
#9958=DIRECTION('center_axis',(0.,-1.,0.));
#9959=DIRECTION('ref_axis',(1.,0.,0.));
#9960=DIRECTION('',(-1.,0.,0.));
#9961=DIRECTION('',(1.,0.,0.));
#9962=DIRECTION('center_axis',(0.,-1.,0.));
#9963=DIRECTION('ref_axis',(1.,0.,0.));
#9964=DIRECTION('',(-1.,0.,0.));
#9965=DIRECTION('',(1.,0.,0.));
#9966=DIRECTION('center_axis',(0.,-1.,0.));
#9967=DIRECTION('ref_axis',(1.,0.,0.));
#9968=DIRECTION('',(-1.,0.,0.));
#9969=DIRECTION('',(1.,0.,0.));
#9970=DIRECTION('center_axis',(0.,-1.,0.));
#9971=DIRECTION('ref_axis',(1.,0.,0.));
#9972=DIRECTION('',(-1.,0.,0.));
#9973=DIRECTION('',(1.,0.,0.));
#9974=DIRECTION('center_axis',(0.,-1.,0.));
#9975=DIRECTION('ref_axis',(1.,0.,0.));
#9976=DIRECTION('',(-1.,0.,0.));
#9977=DIRECTION('',(1.,0.,0.));
#9978=DIRECTION('center_axis',(0.,-1.,0.));
#9979=DIRECTION('ref_axis',(1.,0.,0.));
#9980=DIRECTION('',(-1.,0.,0.));
#9981=DIRECTION('',(1.,0.,0.));
#9982=DIRECTION('center_axis',(0.,-1.,0.));
#9983=DIRECTION('ref_axis',(1.,0.,0.));
#9984=DIRECTION('',(-1.,0.,0.));
#9985=DIRECTION('',(1.,0.,0.));
#9986=DIRECTION('center_axis',(0.,-1.,0.));
#9987=DIRECTION('ref_axis',(1.,0.,0.));
#9988=DIRECTION('',(-1.,0.,0.));
#9989=DIRECTION('',(1.,0.,0.));
#9990=DIRECTION('center_axis',(0.,-1.,0.));
#9991=DIRECTION('ref_axis',(1.,0.,0.));
#9992=DIRECTION('',(-1.,0.,0.));
#9993=DIRECTION('',(1.,0.,0.));
#9994=DIRECTION('center_axis',(0.,-1.,0.));
#9995=DIRECTION('ref_axis',(1.,0.,0.));
#9996=DIRECTION('',(-1.,0.,0.));
#9997=DIRECTION('',(1.,0.,0.));
#9998=DIRECTION('center_axis',(0.,-1.,0.));
#9999=DIRECTION('ref_axis',(1.,0.,0.));
#10000=DIRECTION('',(-1.,0.,0.));
#10001=DIRECTION('',(1.,0.,0.));
#10002=DIRECTION('center_axis',(0.,-1.,0.));
#10003=DIRECTION('ref_axis',(1.,0.,0.));
#10004=DIRECTION('',(-1.,0.,0.));
#10005=DIRECTION('',(1.,0.,0.));
#10006=DIRECTION('center_axis',(0.,-1.,0.));
#10007=DIRECTION('ref_axis',(1.,0.,0.));
#10008=DIRECTION('',(-1.,0.,0.));
#10009=DIRECTION('',(1.,0.,0.));
#10010=DIRECTION('center_axis',(0.,-1.,0.));
#10011=DIRECTION('ref_axis',(1.,0.,0.));
#10012=DIRECTION('',(-1.,0.,0.));
#10013=DIRECTION('',(1.,0.,0.));
#10014=DIRECTION('center_axis',(0.,-1.,0.));
#10015=DIRECTION('ref_axis',(1.,0.,0.));
#10016=DIRECTION('',(-1.,0.,0.));
#10017=DIRECTION('',(1.,0.,0.));
#10018=DIRECTION('center_axis',(0.,-1.,0.));
#10019=DIRECTION('ref_axis',(1.,0.,0.));
#10020=DIRECTION('',(-1.,0.,0.));
#10021=DIRECTION('',(1.,0.,0.));
#10022=DIRECTION('center_axis',(0.,-1.,0.));
#10023=DIRECTION('ref_axis',(1.,0.,0.));
#10024=DIRECTION('',(-1.,0.,0.));
#10025=DIRECTION('',(1.,0.,0.));
#10026=DIRECTION('center_axis',(0.,-1.,0.));
#10027=DIRECTION('ref_axis',(1.,0.,0.));
#10028=DIRECTION('',(-1.,0.,0.));
#10029=DIRECTION('',(1.,0.,0.));
#10030=DIRECTION('center_axis',(0.,-1.,0.));
#10031=DIRECTION('ref_axis',(1.,0.,0.));
#10032=DIRECTION('',(1.,0.,0.));
#10033=DIRECTION('',(-1.,0.,0.));
#10034=DIRECTION('center_axis',(0.,-1.,0.));
#10035=DIRECTION('ref_axis',(1.,0.,0.));
#10036=DIRECTION('',(1.,0.,0.));
#10037=DIRECTION('',(-1.,0.,0.));
#10038=DIRECTION('center_axis',(0.,-1.,0.));
#10039=DIRECTION('ref_axis',(1.,0.,0.));
#10040=DIRECTION('',(1.,0.,0.));
#10041=DIRECTION('',(-1.,0.,0.));
#10042=DIRECTION('center_axis',(0.,-1.,0.));
#10043=DIRECTION('ref_axis',(1.,0.,0.));
#10044=DIRECTION('',(1.,0.,0.));
#10045=DIRECTION('',(-1.,0.,0.));
#10046=DIRECTION('center_axis',(0.,-1.,0.));
#10047=DIRECTION('ref_axis',(1.,0.,0.));
#10048=DIRECTION('',(1.,0.,0.));
#10049=DIRECTION('',(-1.,0.,0.));
#10050=DIRECTION('center_axis',(0.,-1.,0.));
#10051=DIRECTION('ref_axis',(1.,0.,0.));
#10052=DIRECTION('',(1.,0.,0.));
#10053=DIRECTION('',(-1.,0.,0.));
#10054=DIRECTION('center_axis',(0.,-1.,0.));
#10055=DIRECTION('ref_axis',(1.,0.,0.));
#10056=DIRECTION('',(1.,0.,0.));
#10057=DIRECTION('',(-1.,0.,0.));
#10058=DIRECTION('center_axis',(0.,-1.,0.));
#10059=DIRECTION('ref_axis',(1.,0.,0.));
#10060=DIRECTION('',(1.,0.,0.));
#10061=DIRECTION('',(-1.,0.,0.));
#10062=DIRECTION('center_axis',(0.,-1.,0.));
#10063=DIRECTION('ref_axis',(1.,0.,0.));
#10064=DIRECTION('',(1.,0.,0.));
#10065=DIRECTION('',(0.,0.,1.));
#10066=DIRECTION('',(-1.,0.,0.));
#10067=DIRECTION('center_axis',(0.,-1.,0.));
#10068=DIRECTION('ref_axis',(1.,0.,0.));
#10069=DIRECTION('',(1.,0.,0.));
#10070=DIRECTION('',(-1.,0.,0.));
#10071=DIRECTION('center_axis',(0.,-1.,0.));
#10072=DIRECTION('ref_axis',(1.,0.,0.));
#10073=DIRECTION('',(1.,0.,0.));
#10074=DIRECTION('',(-1.,0.,0.));
#10075=DIRECTION('center_axis',(0.,-1.,0.));
#10076=DIRECTION('ref_axis',(1.,0.,0.));
#10077=DIRECTION('',(1.,0.,0.));
#10078=DIRECTION('',(-1.,0.,0.));
#10079=DIRECTION('center_axis',(0.,-1.,0.));
#10080=DIRECTION('ref_axis',(1.,0.,0.));
#10081=DIRECTION('',(1.,0.,0.));
#10082=DIRECTION('',(-1.,0.,0.));
#10083=DIRECTION('center_axis',(0.,-1.,0.));
#10084=DIRECTION('ref_axis',(1.,0.,0.));
#10085=DIRECTION('',(1.,0.,0.));
#10086=DIRECTION('',(-1.,0.,0.));
#10087=DIRECTION('center_axis',(0.,-1.,0.));
#10088=DIRECTION('ref_axis',(1.,0.,0.));
#10089=DIRECTION('',(1.,0.,0.));
#10090=DIRECTION('',(-1.,0.,0.));
#10091=DIRECTION('center_axis',(0.,-1.,0.));
#10092=DIRECTION('ref_axis',(1.,0.,0.));
#10093=DIRECTION('',(1.,0.,0.));
#10094=DIRECTION('',(-1.,0.,0.));
#10095=DIRECTION('center_axis',(0.,-1.,0.));
#10096=DIRECTION('ref_axis',(1.,0.,0.));
#10097=DIRECTION('',(1.,0.,0.));
#10098=DIRECTION('',(-1.,0.,0.));
#10099=DIRECTION('center_axis',(0.,-1.,0.));
#10100=DIRECTION('ref_axis',(1.,0.,0.));
#10101=DIRECTION('',(1.,0.,0.));
#10102=DIRECTION('',(-1.,0.,0.));
#10103=DIRECTION('center_axis',(0.,0.,1.));
#10104=DIRECTION('ref_axis',(1.,0.,0.));
#10105=DIRECTION('',(0.,1.,0.));
#10106=DIRECTION('',(0.994646105081306,0.103339855073382,0.));
#10107=DIRECTION('',(1.,0.,0.));
#10108=DIRECTION('',(0.,-1.,0.));
#10109=DIRECTION('center_axis',(1.,0.,0.));
#10110=DIRECTION('ref_axis',(0.,1.,0.));
#10111=DIRECTION('',(0.,0.,1.));
#10112=DIRECTION('',(0.,1.,0.));
#10113=DIRECTION('center_axis',(1.,0.,0.));
#10114=DIRECTION('ref_axis',(0.,1.,0.));
#10115=DIRECTION('',(0.,0.,1.));
#10116=DIRECTION('',(0.,-1.,0.));
#10117=DIRECTION('',(0.,0.,1.));
#10118=DIRECTION('',(0.,1.,0.));
#10119=DIRECTION('center_axis',(-1.,0.,0.));
#10120=DIRECTION('ref_axis',(0.,-1.,0.));
#10121=DIRECTION('',(0.,-1.,0.));
#10122=DIRECTION('',(0.,0.,1.));
#10123=DIRECTION('center_axis',(-0.103339855073382,0.994646105081306,0.));
#10124=DIRECTION('ref_axis',(-0.994646105081306,-0.103339855073382,0.));
#10125=DIRECTION('',(-0.994646105081306,-0.103339855073382,0.));
#10126=DIRECTION('',(0.,0.,1.));
#10127=DIRECTION('center_axis',(0.,1.,0.));
#10128=DIRECTION('ref_axis',(-1.,0.,0.));
#10129=DIRECTION('',(-1.,0.,0.));
#10130=DIRECTION('',(1.,0.,0.));
#10131=DIRECTION('center_axis',(0.,0.,1.));
#10132=DIRECTION('ref_axis',(1.,0.,0.));
#10133=DIRECTION('center_axis',(0.,0.,1.));
#10134=DIRECTION('ref_axis',(1.,0.,0.));
#10135=DIRECTION('',(-0.447213595499958,-0.894427190999916,0.));
#10136=DIRECTION('',(-0.694594513699567,0.719401460617409,0.));
#10137=DIRECTION('',(-1.,0.,0.));
#10138=DIRECTION('',(0.,1.,0.));
#10139=DIRECTION('',(1.,0.,0.));
#10140=DIRECTION('',(0.87524153543927,-0.483686111690123,0.));
#10141=DIRECTION('center_axis',(0.,0.,1.));
#10142=DIRECTION('ref_axis',(1.,0.,0.));
#10143=DIRECTION('center_axis',(0.,0.,1.));
#10144=DIRECTION('ref_axis',(1.,0.,0.));
#10145=DIRECTION('center_axis',(0.,0.,1.));
#10146=DIRECTION('ref_axis',(1.,0.,0.));
#10147=DIRECTION('',(0.,0.,-1.));
#10148=DIRECTION('center_axis',(-0.483686111690123,-0.87524153543927,0.));
#10149=DIRECTION('ref_axis',(0.87524153543927,-0.483686111690123,0.));
#10150=DIRECTION('',(0.,0.,1.));
#10151=DIRECTION('',(0.,0.,1.));
#10152=DIRECTION('',(0.87524153543927,-0.483686111690123,0.));
#10153=DIRECTION('center_axis',(-0.894427190999916,0.447213595499958,0.));
#10154=DIRECTION('ref_axis',(-0.447213595499958,-0.894427190999916,0.));
#10155=DIRECTION('',(-0.447213595499958,-0.894427190999916,0.));
#10156=DIRECTION('',(0.,0.,1.));
#10157=DIRECTION('center_axis',(0.719401460617409,0.694594513699567,0.));
#10158=DIRECTION('ref_axis',(-0.694594513699567,0.719401460617409,0.));
#10159=DIRECTION('',(-0.694594513699567,0.719401460617409,0.));
#10160=DIRECTION('',(0.,0.,1.));
#10161=DIRECTION('center_axis',(0.,1.,0.));
#10162=DIRECTION('ref_axis',(-1.,0.,0.));
#10163=DIRECTION('',(-1.,0.,0.));
#10164=DIRECTION('',(0.,0.,1.));
#10165=DIRECTION('center_axis',(1.,0.,0.));
#10166=DIRECTION('ref_axis',(0.,1.,0.));
#10167=DIRECTION('',(0.,1.,0.));
#10168=DIRECTION('',(0.,0.,1.));
#10169=DIRECTION('center_axis',(0.,-1.,0.));
#10170=DIRECTION('ref_axis',(1.,0.,0.));
#10171=DIRECTION('',(1.,0.,0.));
#10172=DIRECTION('center_axis',(0.,0.,1.));
#10173=DIRECTION('ref_axis',(1.,0.,0.));
#10174=DIRECTION('center_axis',(0.,0.,1.));
#10175=DIRECTION('ref_axis',(1.,0.,0.));
#10176=DIRECTION('center_axis',(0.,0.,1.));
#10177=DIRECTION('ref_axis',(1.,0.,0.));
#11407=CARTESIAN_POINT('',(0.,0.,0.));
#11408=CARTESIAN_POINT('Origin',(6.,-2.5,0.3));
#11409=CARTESIAN_POINT('',(5.83,-2.5,0.6));
#11410=CARTESIAN_POINT('Origin',(6.,-2.5,0.6));
#11411=CARTESIAN_POINT('',(5.83,-2.5,0.));
#11412=CARTESIAN_POINT('',(5.83,-2.5,0.3));
#11413=CARTESIAN_POINT('Origin',(6.,-2.5,0.));
#11414=CARTESIAN_POINT('Origin',(12.8,-2.5,0.3));
#11415=CARTESIAN_POINT('',(12.63,-2.5,0.6));
#11416=CARTESIAN_POINT('Origin',(12.8,-2.5,0.6));
#11417=CARTESIAN_POINT('',(12.63,-2.5,0.));
#11418=CARTESIAN_POINT('',(12.63,-2.5,0.3));
#11419=CARTESIAN_POINT('Origin',(12.8,-2.5,0.));
#11420=CARTESIAN_POINT('Origin',(0.,0.,0.3));
#11421=CARTESIAN_POINT('',(-0.41,5.02105187650415E-17,0.6));
#11422=CARTESIAN_POINT('Origin',(0.,0.,0.6));
#11423=CARTESIAN_POINT('',(-0.41,5.02105187650415E-17,0.));
#11424=CARTESIAN_POINT('',(-0.41,5.02105187650415E-17,0.3));
#11425=CARTESIAN_POINT('Origin',(0.,0.,0.));
#11426=CARTESIAN_POINT('Origin',(-3.,0.08,0.6));
#11427=CARTESIAN_POINT('',(-2.94222222222222,0.,0.6));
#11428=CARTESIAN_POINT('',(-2.94222222222222,0.,-0.3));
#11429=CARTESIAN_POINT('',(-2.94222222222222,-2.22044604925031E-16,0.3));
#11430=CARTESIAN_POINT('',(-3.,0.08,0.6));
#11431=CARTESIAN_POINT('',(-2.4668154158215,-0.658255578093306,0.6));
#11432=CARTESIAN_POINT('',(-3.,0.08,-0.3));
#11433=CARTESIAN_POINT('',(-3.,0.08,0.6));
#11434=CARTESIAN_POINT('',(-3.62244421906694,0.94184584178499,-0.3));
#11435=CARTESIAN_POINT('Origin',(-3.065,-0.01,0.6));
#11436=CARTESIAN_POINT('',(-3.05777777777778,0.,-0.3));
#11437=CARTESIAN_POINT('',(-3.05777777777778,0.,0.6));
#11438=CARTESIAN_POINT('',(-3.05777777777778,4.44089209850063E-16,0.3));
#11439=CARTESIAN_POINT('',(-3.45559330628803,-0.550821501014198,-0.3));
#11440=CARTESIAN_POINT('',(-2.53728701825558,0.720679513184584,0.6));
#11441=CARTESIAN_POINT('Origin',(-3.4,0.08,0.6));
#11442=CARTESIAN_POINT('',(-3.34222222222222,0.,0.6));
#11443=CARTESIAN_POINT('',(-3.34222222222222,0.,-0.3));
#11444=CARTESIAN_POINT('',(-3.34222222222222,-2.22044604925031E-16,0.3));
#11445=CARTESIAN_POINT('',(-3.4,0.08,0.6));
#11446=CARTESIAN_POINT('',(-2.79825557809331,-0.753184584178499,0.6));
#11447=CARTESIAN_POINT('',(-3.4,0.08,-0.3));
#11448=CARTESIAN_POINT('',(-3.4,0.08,0.6));
#11449=CARTESIAN_POINT('',(-3.95388438133874,0.846916835699797,-0.3));
#11450=CARTESIAN_POINT('Origin',(-3.465,-0.01,0.6));
#11451=CARTESIAN_POINT('',(-3.45777777777778,0.,-0.3));
#11452=CARTESIAN_POINT('',(-3.45777777777778,0.,0.6));
#11453=CARTESIAN_POINT('',(-3.45777777777778,2.22044604925031E-16,0.3));
#11454=CARTESIAN_POINT('',(-3.78703346855984,-0.455892494929006,-0.3));
#11455=CARTESIAN_POINT('',(-2.86872718052738,0.815608519269777,0.6));
#11456=CARTESIAN_POINT('Origin',(-3.8,0.08,0.6));
#11457=CARTESIAN_POINT('',(-3.74222222222222,0.,0.6));
#11458=CARTESIAN_POINT('',(-3.74222222222222,0.,-0.3));
#11459=CARTESIAN_POINT('',(-3.74222222222222,2.22044604925031E-16,0.3));
#11460=CARTESIAN_POINT('',(-3.8,0.08,0.6));
#11461=CARTESIAN_POINT('',(-3.12969574036512,-0.84811359026369,0.6));
#11462=CARTESIAN_POINT('',(-3.8,0.08,-0.3));
#11463=CARTESIAN_POINT('',(-3.8,0.08,0.6));
#11464=CARTESIAN_POINT('',(-4.28532454361054,0.751987829614604,-0.3));
#11465=CARTESIAN_POINT('Origin',(-3.865,-0.01,0.6));
#11466=CARTESIAN_POINT('',(-3.85777777777778,0.,-0.3));
#11467=CARTESIAN_POINT('',(-3.85777777777778,0.,0.6));
#11468=CARTESIAN_POINT('',(-3.85777777777778,4.44089209850063E-16,0.3));
#11469=CARTESIAN_POINT('',(-4.11847363083164,-0.360963488843813,-0.3));
#11470=CARTESIAN_POINT('',(-3.20016734279919,0.910537525354969,0.6));
#11471=CARTESIAN_POINT('Origin',(-4.2,0.08,0.6));
#11472=CARTESIAN_POINT('',(-4.14222222222222,0.,0.6));
#11473=CARTESIAN_POINT('',(-4.14222222222222,0.,-0.3));
#11474=CARTESIAN_POINT('',(-4.14222222222222,0.,0.3));
#11475=CARTESIAN_POINT('',(-4.2,0.08,0.6));
#11476=CARTESIAN_POINT('',(-3.46113590263691,-0.943042596348886,0.6));
#11477=CARTESIAN_POINT('',(-4.2,0.08,-0.3));
#11478=CARTESIAN_POINT('',(-4.2,0.08,0.6));
#11479=CARTESIAN_POINT('',(-4.61676470588236,0.657058823529412,-0.3));
#11480=CARTESIAN_POINT('Origin',(-4.265,-0.01,0.6));
#11481=CARTESIAN_POINT('',(-4.25777777777778,0.,-0.3));
#11482=CARTESIAN_POINT('',(-4.25777777777778,0.,0.6));
#11483=CARTESIAN_POINT('',(-4.25777777777778,-2.22044604925031E-16,0.3));
#11484=CARTESIAN_POINT('',(-4.44991379310344,-0.266034482758619,-0.3));
#11485=CARTESIAN_POINT('',(-3.531607505071,1.00546653144016,0.6));
#11486=CARTESIAN_POINT('Origin',(-4.6,0.08,0.6));
#11487=CARTESIAN_POINT('',(-4.54222222222222,0.,0.6));
#11488=CARTESIAN_POINT('',(-4.54222222222222,0.,-0.3));
#11489=CARTESIAN_POINT('',(-4.54222222222222,2.22044604925031E-16,0.3));
#11490=CARTESIAN_POINT('',(-4.6,0.08,0.6));
#11491=CARTESIAN_POINT('',(-3.79257606490873,-1.03797160243407,0.6));
#11492=CARTESIAN_POINT('',(-4.6,0.08,-0.3));
#11493=CARTESIAN_POINT('',(-4.6,0.08,0.6));
#11494=CARTESIAN_POINT('',(-4.94820486815415,0.562129817444219,-0.3));
#11495=CARTESIAN_POINT('Origin',(-4.665,-0.01,0.6));
#11496=CARTESIAN_POINT('',(-4.65777777777778,0.,-0.3));
#11497=CARTESIAN_POINT('',(-4.65777777777778,0.,0.6));
#11498=CARTESIAN_POINT('',(-4.65777777777778,0.,0.3));
#11499=CARTESIAN_POINT('',(-4.78135395537526,-0.171105476673429,-0.3));
#11500=CARTESIAN_POINT('',(-3.86304766734279,1.10039553752536,0.6));
#11501=CARTESIAN_POINT('Origin',(-5.,0.08,0.6));
#11502=CARTESIAN_POINT('',(-4.94222222222222,0.,0.6));
#11503=CARTESIAN_POINT('',(-4.94222222222222,0.,-0.3));
#11504=CARTESIAN_POINT('',(-4.94222222222222,0.,0.3));
#11505=CARTESIAN_POINT('',(-5.,0.08,0.6));
#11506=CARTESIAN_POINT('',(-4.12401622718054,-1.13290060851927,0.6));
#11507=CARTESIAN_POINT('',(-5.,0.08,-0.3));
#11508=CARTESIAN_POINT('',(-5.,0.08,0.6));
#11509=CARTESIAN_POINT('',(-5.27964503042596,0.467200811359026,-0.3));
#11510=CARTESIAN_POINT('Origin',(-5.065,-0.01,0.6));
#11511=CARTESIAN_POINT('',(-5.05777777777778,0.,-0.3));
#11512=CARTESIAN_POINT('',(-5.05777777777778,0.,0.6));
#11513=CARTESIAN_POINT('',(-5.05777777777778,-2.22044604925031E-16,0.3));
#11514=CARTESIAN_POINT('',(-5.11279411764706,-0.076176470588234,-0.3));
#11515=CARTESIAN_POINT('',(-4.19448782961461,1.19532454361054,0.6));
#11516=CARTESIAN_POINT('Origin',(-5.4,0.08,0.6));
#11517=CARTESIAN_POINT('',(-5.34222222222222,0.,0.6));
#11518=CARTESIAN_POINT('',(-5.34222222222222,0.,-0.3));
#11519=CARTESIAN_POINT('',(-5.34222222222222,0.,0.3));
#11520=CARTESIAN_POINT('',(-5.4,0.08,0.6));
#11521=CARTESIAN_POINT('',(-4.45545638945233,-1.22782961460446,0.6));
#11522=CARTESIAN_POINT('',(-5.4,0.08,-0.3));
#11523=CARTESIAN_POINT('',(-5.4,0.08,0.6));
#11524=CARTESIAN_POINT('',(-5.61108519269777,0.372271805273833,-0.3));
#11525=CARTESIAN_POINT('Origin',(-5.465,-0.01,0.6));
#11526=CARTESIAN_POINT('',(-5.45777777777778,0.,-0.3));
#11527=CARTESIAN_POINT('',(-5.45777777777778,0.,0.6));
#11528=CARTESIAN_POINT('',(-5.45777777777778,-2.22044604925031E-16,0.3));
#11529=CARTESIAN_POINT('',(-5.44423427991886,0.0187525354969586,-0.3));
#11530=CARTESIAN_POINT('',(-4.52592799188642,1.29025354969574,0.6));
#11531=CARTESIAN_POINT('Origin',(-5.8,0.08,0.6));
#11532=CARTESIAN_POINT('',(-5.74222222222222,0.,0.6));
#11533=CARTESIAN_POINT('',(-5.74222222222222,0.,-0.3));
#11534=CARTESIAN_POINT('',(-5.74222222222222,2.22044604925031E-16,0.3));
#11535=CARTESIAN_POINT('',(-5.8,0.08,0.6));
#11536=CARTESIAN_POINT('',(-4.78689655172415,-1.32275862068965,0.6));
#11537=CARTESIAN_POINT('',(-5.8,0.08,-0.3));
#11538=CARTESIAN_POINT('',(-5.8,0.08,0.6));
#11539=CARTESIAN_POINT('',(-5.94252535496957,0.277342799188642,-0.3));
#11540=CARTESIAN_POINT('Origin',(-5.865,-0.01,0.6));
#11541=CARTESIAN_POINT('',(-5.85777777777778,0.,-0.3));
#11542=CARTESIAN_POINT('',(-5.85777777777778,0.,0.6));
#11543=CARTESIAN_POINT('',(-5.85777777777778,0.,0.3));
#11544=CARTESIAN_POINT('',(-5.77567444219067,0.113681541582149,-0.3));
#11545=CARTESIAN_POINT('',(-4.85736815415821,1.38518255578094,0.6));
#11546=CARTESIAN_POINT('Origin',(-6.2,0.08,0.6));
#11547=CARTESIAN_POINT('',(-6.14222222222222,0.,0.6));
#11548=CARTESIAN_POINT('',(-6.14222222222222,0.,-0.3));
#11549=CARTESIAN_POINT('',(-6.14222222222222,2.22044604925031E-16,0.3));
#11550=CARTESIAN_POINT('',(-6.2,0.08,0.6));
#11551=CARTESIAN_POINT('',(-5.11833671399593,-1.41768762677485,0.6));
#11552=CARTESIAN_POINT('',(-6.2,0.08,-0.3));
#11553=CARTESIAN_POINT('',(-6.2,0.08,0.6));
#11554=CARTESIAN_POINT('',(-6.27396551724138,0.182413793103448,-0.3));
#11555=CARTESIAN_POINT('Origin',(-6.265,-0.01,0.6));
#11556=CARTESIAN_POINT('',(-6.25777777777778,0.,-0.3));
#11557=CARTESIAN_POINT('',(-6.25777777777778,0.,0.6));
#11558=CARTESIAN_POINT('',(-6.25777777777778,-2.22044604925031E-16,0.3));
#11559=CARTESIAN_POINT('',(-6.10711460446247,0.208610547667344,-0.3));
#11560=CARTESIAN_POINT('',(-5.18880831643003,1.48011156186612,0.6));
#11561=CARTESIAN_POINT('Origin',(-10.2,0.08,0.6));
#11562=CARTESIAN_POINT('',(-10.1422222222222,0.,0.6));
#11563=CARTESIAN_POINT('',(-10.1422222222222,0.,-0.3));
#11564=CARTESIAN_POINT('',(-10.1422222222222,1.38777878078145E-17,0.3));
#11565=CARTESIAN_POINT('',(-10.2,0.08,0.6));
#11566=CARTESIAN_POINT('',(-8.43273833671401,-2.36697768762677,0.6));
#11567=CARTESIAN_POINT('',(-10.2,0.08,-0.3));
#11568=CARTESIAN_POINT('',(-10.2,0.08,0.6));
#11569=CARTESIAN_POINT('',(-9.58836713995944,-0.766876267748476,-0.3));
#11570=CARTESIAN_POINT('Origin',(-10.265,-0.01,0.6));
#11571=CARTESIAN_POINT('',(-10.2577777777778,0.,-0.3));
#11572=CARTESIAN_POINT('',(-10.2577777777778,0.,0.6));
#11573=CARTESIAN_POINT('',(-10.2577777777778,6.93889390390723E-18,0.3));
#11574=CARTESIAN_POINT('',(-9.42151622718051,1.15790060851927,-0.3));
#11575=CARTESIAN_POINT('',(-8.50320993914803,2.42940162271807,0.6));
#11576=CARTESIAN_POINT('Origin',(-6.8,0.08,0.6));
#11577=CARTESIAN_POINT('',(-6.74222222222222,0.,0.6));
#11578=CARTESIAN_POINT('',(-6.74222222222222,0.,-0.3));
#11579=CARTESIAN_POINT('',(-6.74222222222222,1.11022302462516E-16,0.3));
#11580=CARTESIAN_POINT('',(-6.8,0.08,0.6));
#11581=CARTESIAN_POINT('',(-5.61549695740364,-1.56008113590264,0.6));
#11582=CARTESIAN_POINT('',(-6.8,0.08,-0.3));
#11583=CARTESIAN_POINT('',(-6.8,0.08,0.6));
#11584=CARTESIAN_POINT('',(-6.77112576064909,0.0400202839756583,-0.3));
#11585=CARTESIAN_POINT('Origin',(-6.865,-0.01,0.6));
#11586=CARTESIAN_POINT('',(-6.85777777777778,0.,-0.3));
#11587=CARTESIAN_POINT('',(-6.85777777777778,0.,0.6));
#11588=CARTESIAN_POINT('',(-6.85777777777778,1.11022302462516E-16,0.3));
#11589=CARTESIAN_POINT('',(-6.60427484787018,0.351004056795132,-0.3));
#11590=CARTESIAN_POINT('',(-5.68596855983772,1.62250507099392,0.6));
#11591=CARTESIAN_POINT('Origin',(-7.2,0.08,0.6));
#11592=CARTESIAN_POINT('',(-7.14222222222222,0.,0.6));
#11593=CARTESIAN_POINT('',(-7.14222222222222,0.,-0.3));
#11594=CARTESIAN_POINT('',(-7.14222222222222,1.11022302462516E-16,0.3));
#11595=CARTESIAN_POINT('',(-7.2,0.08,0.6));
#11596=CARTESIAN_POINT('',(-5.94693711967545,-1.65501014198783,0.6));
#11597=CARTESIAN_POINT('',(-7.2,0.08,-0.3));
#11598=CARTESIAN_POINT('',(-7.2,0.08,0.6));
#11599=CARTESIAN_POINT('',(-7.10256592292089,-0.0549087221095346,-0.3));
#11600=CARTESIAN_POINT('Origin',(-7.265,-0.01,0.6));
#11601=CARTESIAN_POINT('',(-7.25777777777778,0.,-0.3));
#11602=CARTESIAN_POINT('',(-7.25777777777778,0.,0.6));
#11603=CARTESIAN_POINT('',(-7.25777777777778,1.11022302462516E-16,0.3));
#11604=CARTESIAN_POINT('',(-6.93571501014199,0.445933062880325,-0.3));
#11605=CARTESIAN_POINT('',(-6.01740872210952,1.71743407707911,0.6));
#11606=CARTESIAN_POINT('Origin',(-7.6,0.08,0.6));
#11607=CARTESIAN_POINT('',(-7.54222222222222,0.,0.6));
#11608=CARTESIAN_POINT('',(-7.54222222222222,0.,-0.3));
#11609=CARTESIAN_POINT('',(-7.54222222222222,0.,0.3));
#11610=CARTESIAN_POINT('',(-7.6,0.08,0.6));
#11611=CARTESIAN_POINT('',(-6.27837728194725,-1.74993914807303,0.6));
#11612=CARTESIAN_POINT('',(-7.6,0.08,-0.3));
#11613=CARTESIAN_POINT('',(-7.6,0.08,0.6));
#11614=CARTESIAN_POINT('',(-7.43400608519269,-0.149837728194727,-0.3));
#11615=CARTESIAN_POINT('Origin',(-7.665,-0.01,0.6));
#11616=CARTESIAN_POINT('',(-7.65777777777778,0.,-0.3));
#11617=CARTESIAN_POINT('',(-7.65777777777778,0.,0.6));
#11618=CARTESIAN_POINT('',(-7.65777777777778,1.11022302462516E-16,0.3));
#11619=CARTESIAN_POINT('',(-7.26715517241379,0.540862068965518,-0.3));
#11620=CARTESIAN_POINT('',(-6.34884888438131,1.81236308316431,0.6));
#11621=CARTESIAN_POINT('Origin',(-8.,0.08,0.6));
#11622=CARTESIAN_POINT('',(-7.94222222222222,0.,0.6));
#11623=CARTESIAN_POINT('',(-7.94222222222222,0.,-0.3));
#11624=CARTESIAN_POINT('',(-7.94222222222222,0.,0.3));
#11625=CARTESIAN_POINT('',(-8.,0.08,0.6));
#11626=CARTESIAN_POINT('',(-6.60981744421906,-1.84486815415822,0.6));
#11627=CARTESIAN_POINT('',(-8.,0.08,-0.3));
#11628=CARTESIAN_POINT('',(-8.,0.08,0.6));
#11629=CARTESIAN_POINT('',(-7.7654462474645,-0.24476673427992,-0.3));
#11630=CARTESIAN_POINT('Origin',(-8.065,-0.01,0.6));
#11631=CARTESIAN_POINT('',(-8.05777777777778,0.,-0.3));
#11632=CARTESIAN_POINT('',(-8.05777777777778,0.,0.6));
#11633=CARTESIAN_POINT('',(-8.05777777777778,1.11022302462516E-16,0.3));
#11634=CARTESIAN_POINT('',(-7.59859533468559,0.635791075050711,-0.3));
#11635=CARTESIAN_POINT('',(-6.68028904665311,1.90729208924951,0.6));
#11636=CARTESIAN_POINT('Origin',(-8.4,0.08,0.6));
#11637=CARTESIAN_POINT('',(-8.34222222222222,0.,0.6));
#11638=CARTESIAN_POINT('',(-8.34222222222222,0.,-0.3));
#11639=CARTESIAN_POINT('',(-8.34222222222222,0.,0.3));
#11640=CARTESIAN_POINT('',(-8.4,0.08,0.6));
#11641=CARTESIAN_POINT('',(-6.94125760649083,-1.93979716024342,0.6));
#11642=CARTESIAN_POINT('',(-8.4,0.08,-0.3));
#11643=CARTESIAN_POINT('',(-8.4,0.08,0.6));
#11644=CARTESIAN_POINT('',(-8.0968864097363,-0.339695740365117,-0.3));
#11645=CARTESIAN_POINT('Origin',(-8.465,-0.01,0.6));
#11646=CARTESIAN_POINT('',(-8.45777777777778,0.,-0.3));
#11647=CARTESIAN_POINT('',(-8.45777777777778,0.,0.6));
#11648=CARTESIAN_POINT('',(-8.45777777777778,0.,0.3));
#11649=CARTESIAN_POINT('',(-7.93003549695741,0.730720081135902,-0.3));
#11650=CARTESIAN_POINT('',(-7.01172920892496,2.00222109533468,0.6));
#11651=CARTESIAN_POINT('Origin',(-8.8,0.08,0.6));
#11652=CARTESIAN_POINT('',(-8.74222222222222,0.,0.6));
#11653=CARTESIAN_POINT('',(-8.74222222222222,0.,-0.3));
#11654=CARTESIAN_POINT('',(-8.74222222222222,0.,0.3));
#11655=CARTESIAN_POINT('',(-8.8,0.08,0.6));
#11656=CARTESIAN_POINT('',(-7.27269776876264,-2.03472616632861,0.6));
#11657=CARTESIAN_POINT('',(-8.8,0.08,-0.3));
#11658=CARTESIAN_POINT('',(-8.8,0.08,0.6));
#11659=CARTESIAN_POINT('',(-8.4283265720081,-0.43462474645031,-0.3));
#11660=CARTESIAN_POINT('Origin',(-8.865,-0.01,0.6));
#11661=CARTESIAN_POINT('',(-8.85777777777778,0.,-0.3));
#11662=CARTESIAN_POINT('',(-8.85777777777778,0.,0.6));
#11663=CARTESIAN_POINT('',(-8.85777777777778,-5.55111512312578E-17,0.3));
#11664=CARTESIAN_POINT('',(-8.26147565922921,0.825649087221095,-0.3));
#11665=CARTESIAN_POINT('',(-7.34316937119677,2.09715010141987,0.6));
#11666=CARTESIAN_POINT('Origin',(-9.2,0.08,0.6));
#11667=CARTESIAN_POINT('',(-9.14222222222222,0.,0.6));
#11668=CARTESIAN_POINT('',(-9.14222222222222,0.,-0.3));
#11669=CARTESIAN_POINT('',(-9.14222222222222,0.,0.3));
#11670=CARTESIAN_POINT('',(-9.2,0.08,0.6));
#11671=CARTESIAN_POINT('',(-7.6041379310345,-2.12965517241379,0.6));
#11672=CARTESIAN_POINT('',(-9.2,0.08,-0.3));
#11673=CARTESIAN_POINT('',(-9.2,0.08,0.6));
#11674=CARTESIAN_POINT('',(-8.75976673427992,-0.529553752535495,-0.3));
#11675=CARTESIAN_POINT('Origin',(-9.265,-0.01,0.6));
#11676=CARTESIAN_POINT('',(-9.25777777777778,0.,-0.3));
#11677=CARTESIAN_POINT('',(-9.25777777777778,0.,0.6));
#11678=CARTESIAN_POINT('',(-9.25777777777778,0.,0.3));
#11679=CARTESIAN_POINT('',(-8.592915821501,0.920578093306291,-0.3));
#11680=CARTESIAN_POINT('',(-7.67460953346852,2.19207910750508,0.6));
#11681=CARTESIAN_POINT('Origin',(-9.6,0.08,0.6));
#11682=CARTESIAN_POINT('',(-9.54222222222222,0.,0.6));
#11683=CARTESIAN_POINT('',(-9.54222222222222,0.,-0.3));
#11684=CARTESIAN_POINT('',(-9.54222222222222,0.,0.3));
#11685=CARTESIAN_POINT('',(-9.6,0.08,0.6));
#11686=CARTESIAN_POINT('',(-7.9355780933063,-2.22458417849898,0.6));
#11687=CARTESIAN_POINT('',(-9.6,0.08,-0.3));
#11688=CARTESIAN_POINT('',(-9.6,0.08,0.6));
#11689=CARTESIAN_POINT('',(-9.09120689655173,-0.624482758620687,-0.3));
#11690=CARTESIAN_POINT('Origin',(-9.665,-0.01,0.6));
#11691=CARTESIAN_POINT('',(-9.65777777777778,0.,-0.3));
#11692=CARTESIAN_POINT('',(-9.65777777777778,0.,0.6));
#11693=CARTESIAN_POINT('',(-9.65777777777778,-2.77555756156289E-17,0.3));
#11694=CARTESIAN_POINT('',(-8.9243559837728,1.01550709939148,-0.3));
#11695=CARTESIAN_POINT('',(-8.00604969574032,2.28700811359028,0.6));
#11696=CARTESIAN_POINT('Origin',(-10.,0.08,0.6));
#11697=CARTESIAN_POINT('',(-9.94222222222222,0.,0.6));
#11698=CARTESIAN_POINT('',(-9.94222222222222,0.,-0.3));
#11699=CARTESIAN_POINT('',(-9.94222222222222,0.,0.3));
#11700=CARTESIAN_POINT('',(-10.,0.08,0.6));
#11701=CARTESIAN_POINT('',(-8.26701825557805,-2.31951318458419,0.6));
#11702=CARTESIAN_POINT('',(-10.,0.08,-0.3));
#11703=CARTESIAN_POINT('',(-10.,0.08,0.6));
#11704=CARTESIAN_POINT('',(-9.42264705882351,-0.71941176470589,-0.3));
#11705=CARTESIAN_POINT('Origin',(-10.065,-0.01,0.6));
#11706=CARTESIAN_POINT('',(-10.0577777777778,0.,-0.3));
#11707=CARTESIAN_POINT('',(-10.0577777777778,0.,0.6));
#11708=CARTESIAN_POINT('',(-10.0577777777778,0.,0.3));
#11709=CARTESIAN_POINT('',(-9.25579614604461,1.11043610547668,-0.3));
#11710=CARTESIAN_POINT('',(-8.33748985801213,2.38193711967547,0.6));
#11711=CARTESIAN_POINT('Origin',(-9.8,0.08,0.6));
#11712=CARTESIAN_POINT('',(-9.74222222222222,0.,0.6));
#11713=CARTESIAN_POINT('',(-9.74222222222222,0.,-0.3));
#11714=CARTESIAN_POINT('',(-9.74222222222222,2.77555756156289E-17,0.3));
#11715=CARTESIAN_POINT('',(-9.8,0.08,0.6));
#11716=CARTESIAN_POINT('',(-8.10129817444215,-2.2720486815416,0.6));
#11717=CARTESIAN_POINT('',(-9.8,0.08,-0.3));
#11718=CARTESIAN_POINT('',(-9.8,0.08,0.6));
#11719=CARTESIAN_POINT('',(-9.25692697768761,-0.671947261663294,-0.3));
#11720=CARTESIAN_POINT('Origin',(-9.865,-0.01,0.6));
#11721=CARTESIAN_POINT('',(-9.85777777777778,0.,-0.3));
#11722=CARTESIAN_POINT('',(-9.85777777777778,0.,0.6));
#11723=CARTESIAN_POINT('',(-9.85777777777778,-2.77555756156289E-17,0.3));
#11724=CARTESIAN_POINT('',(-9.09007606490873,1.06297160243408,-0.3));
#11725=CARTESIAN_POINT('',(-8.17176977687629,2.33447261663285,0.6));
#11726=CARTESIAN_POINT('Origin',(-9.4,0.08,0.6));
#11727=CARTESIAN_POINT('',(-9.34222222222222,0.,0.6));
#11728=CARTESIAN_POINT('',(-9.34222222222222,0.,-0.3));
#11729=CARTESIAN_POINT('',(-9.34222222222222,0.,0.3));
#11730=CARTESIAN_POINT('',(-9.4,0.08,0.6));
#11731=CARTESIAN_POINT('',(-7.76985801217034,-2.1771196754564,0.6));
#11732=CARTESIAN_POINT('',(-9.4,0.08,-0.3));
#11733=CARTESIAN_POINT('',(-9.4,0.08,0.6));
#11734=CARTESIAN_POINT('',(-8.92548681541581,-0.5770182555781,-0.3));
#11735=CARTESIAN_POINT('Origin',(-9.465,-0.01,0.6));
#11736=CARTESIAN_POINT('',(-9.45777777777778,0.,-0.3));
#11737=CARTESIAN_POINT('',(-9.45777777777778,0.,0.6));
#11738=CARTESIAN_POINT('',(-9.45777777777778,0.,0.3));
#11739=CARTESIAN_POINT('',(-8.75863590263692,0.968042596348883,-0.3));
#11740=CARTESIAN_POINT('',(-7.84032961460448,2.23954361054766,0.6));
#11741=CARTESIAN_POINT('Origin',(-9.,0.08,0.6));
#11742=CARTESIAN_POINT('',(-8.94222222222222,0.,0.6));
#11743=CARTESIAN_POINT('',(-8.94222222222222,0.,-0.3));
#11744=CARTESIAN_POINT('',(-8.94222222222222,0.,0.3));
#11745=CARTESIAN_POINT('',(-9.,0.08,0.6));
#11746=CARTESIAN_POINT('',(-7.43841784989854,-2.08219066937121,0.6));
#11747=CARTESIAN_POINT('',(-9.,0.08,-0.3));
#11748=CARTESIAN_POINT('',(-9.,0.08,0.6));
#11749=CARTESIAN_POINT('',(-8.59404665314401,-0.482089249492907,-0.3));
#11750=CARTESIAN_POINT('Origin',(-9.065,-0.01,0.6));
#11751=CARTESIAN_POINT('',(-9.05777777777778,0.,-0.3));
#11752=CARTESIAN_POINT('',(-9.05777777777778,0.,0.6));
#11753=CARTESIAN_POINT('',(-9.05777777777778,0.,0.3));
#11754=CARTESIAN_POINT('',(-8.4271957403651,0.873113590263694,-0.3));
#11755=CARTESIAN_POINT('',(-7.50888945233262,2.14461460446249,0.6));
#11756=CARTESIAN_POINT('Origin',(-8.6,0.08,0.6));
#11757=CARTESIAN_POINT('',(-8.54222222222222,0.,0.6));
#11758=CARTESIAN_POINT('',(-8.54222222222222,0.,-0.3));
#11759=CARTESIAN_POINT('',(-8.54222222222222,0.,0.3));
#11760=CARTESIAN_POINT('',(-8.6,0.08,0.6));
#11761=CARTESIAN_POINT('',(-7.10697768762679,-1.987261663286,0.6));
#11762=CARTESIAN_POINT('',(-8.6,0.08,-0.3));
#11763=CARTESIAN_POINT('',(-8.6,0.08,0.6));
#11764=CARTESIAN_POINT('',(-8.26260649087221,-0.387160243407706,-0.3));
#11765=CARTESIAN_POINT('Origin',(-8.665,-0.01,0.6));
#11766=CARTESIAN_POINT('',(-8.65777777777778,0.,-0.3));
#11767=CARTESIAN_POINT('',(-8.65777777777778,0.,0.6));
#11768=CARTESIAN_POINT('',(-8.65777777777778,0.,0.3));
#11769=CARTESIAN_POINT('',(-8.09575557809329,0.778184584178501,-0.3));
#11770=CARTESIAN_POINT('',(-7.17744929006081,2.0496855983773,0.6));
#11771=CARTESIAN_POINT('Origin',(-8.2,0.08,0.6));
#11772=CARTESIAN_POINT('',(-8.14222222222222,0.,0.6));
#11773=CARTESIAN_POINT('',(-8.14222222222222,0.,-0.3));
#11774=CARTESIAN_POINT('',(-8.14222222222222,1.11022302462516E-16,0.3));
#11775=CARTESIAN_POINT('',(-8.2,0.08,0.6));
#11776=CARTESIAN_POINT('',(-6.77553752535498,-1.89233265720081,0.6));
#11777=CARTESIAN_POINT('',(-8.2,0.08,-0.3));
#11778=CARTESIAN_POINT('',(-8.2,0.08,0.6));
#11779=CARTESIAN_POINT('',(-7.93116632860041,-0.292231237322513,-0.3));
#11780=CARTESIAN_POINT('Origin',(-8.265,-0.01,0.6));
#11781=CARTESIAN_POINT('',(-8.25777777777778,0.,-0.3));
#11782=CARTESIAN_POINT('',(-8.25777777777778,0.,0.6));
#11783=CARTESIAN_POINT('',(-8.25777777777778,0.,0.3));
#11784=CARTESIAN_POINT('',(-7.76431541582149,0.683255578093308,-0.3));
#11785=CARTESIAN_POINT('',(-6.84600912778901,1.9547565922921,0.6));
#11786=CARTESIAN_POINT('Origin',(-7.8,0.08,0.6));
#11787=CARTESIAN_POINT('',(-7.74222222222222,0.,0.6));
#11788=CARTESIAN_POINT('',(-7.74222222222222,0.,-0.3));
#11789=CARTESIAN_POINT('',(-7.74222222222222,0.,0.3));
#11790=CARTESIAN_POINT('',(-7.8,0.08,0.6));
#11791=CARTESIAN_POINT('',(-6.44409736308315,-1.79740365111562,0.6));
#11792=CARTESIAN_POINT('',(-7.8,0.08,-0.3));
#11793=CARTESIAN_POINT('',(-7.8,0.08,0.6));
#11794=CARTESIAN_POINT('',(-7.5997261663286,-0.197302231237324,-0.3));
#11795=CARTESIAN_POINT('Origin',(-7.865,-0.01,0.6));
#11796=CARTESIAN_POINT('',(-7.85777777777778,0.,-0.3));
#11797=CARTESIAN_POINT('',(-7.85777777777778,0.,0.6));
#11798=CARTESIAN_POINT('',(-7.85777777777778,0.,0.3));
#11799=CARTESIAN_POINT('',(-7.43287525354969,0.588326572008114,-0.3));
#11800=CARTESIAN_POINT('',(-6.51456896551723,1.8598275862069,0.6));
#11801=CARTESIAN_POINT('Origin',(-7.4,0.08,0.6));
#11802=CARTESIAN_POINT('',(-7.34222222222222,0.,0.6));
#11803=CARTESIAN_POINT('',(-7.34222222222222,0.,-0.3));
#11804=CARTESIAN_POINT('',(-7.34222222222222,0.,0.3));
#11805=CARTESIAN_POINT('',(-7.4,0.08,0.6));
#11806=CARTESIAN_POINT('',(-6.11265720081133,-1.70247464503044,0.6));
#11807=CARTESIAN_POINT('',(-7.4,0.08,-0.3));
#11808=CARTESIAN_POINT('',(-7.4,0.08,0.6));
#11809=CARTESIAN_POINT('',(-7.26828600405679,-0.102373225152134,-0.3));
#11810=CARTESIAN_POINT('Origin',(-7.465,-0.01,0.6));
#11811=CARTESIAN_POINT('',(-7.45777777777778,0.,-0.3));
#11812=CARTESIAN_POINT('',(-7.45777777777778,0.,0.6));
#11813=CARTESIAN_POINT('',(-7.45777777777778,-1.11022302462516E-16,0.3));
#11814=CARTESIAN_POINT('',(-7.10143509127789,0.493397565922921,-0.3));
#11815=CARTESIAN_POINT('',(-6.18312880324543,1.76489858012171,0.6));
#11816=CARTESIAN_POINT('Origin',(-7.,0.08,0.6));
#11817=CARTESIAN_POINT('',(-6.94222222222222,0.,0.6));
#11818=CARTESIAN_POINT('',(-6.94222222222222,0.,-0.3));
#11819=CARTESIAN_POINT('',(-6.94222222222222,0.,0.3));
#11820=CARTESIAN_POINT('',(-7.,0.08,0.6));
#11821=CARTESIAN_POINT('',(-5.78121703853954,-1.60754563894524,0.6));
#11822=CARTESIAN_POINT('',(-7.,0.08,-0.3));
#11823=CARTESIAN_POINT('',(-7.,0.08,0.6));
#11824=CARTESIAN_POINT('',(-6.93684584178499,-0.00744421906693815,-0.3));
#11825=CARTESIAN_POINT('Origin',(-7.065,-0.01,0.6));
#11826=CARTESIAN_POINT('',(-7.05777777777778,0.,-0.3));
#11827=CARTESIAN_POINT('',(-7.05777777777778,0.,0.6));
#11828=CARTESIAN_POINT('',(-7.05777777777778,-1.11022302462516E-16,0.3));
#11829=CARTESIAN_POINT('',(-6.76999492900608,0.398468559837728,-0.3));
#11830=CARTESIAN_POINT('',(-5.85168864097362,1.66996957403651,0.6));
#11831=CARTESIAN_POINT('Origin',(-6.6,0.08,0.6));
#11832=CARTESIAN_POINT('',(-6.54222222222222,0.,0.6));
#11833=CARTESIAN_POINT('',(-6.54222222222222,0.,-0.3));
#11834=CARTESIAN_POINT('',(-6.54222222222222,0.,0.3));
#11835=CARTESIAN_POINT('',(-6.6,0.08,0.6));
#11836=CARTESIAN_POINT('',(-5.44977687626774,-1.51261663286004,0.6));
#11837=CARTESIAN_POINT('',(-6.6,0.08,-0.3));
#11838=CARTESIAN_POINT('',(-6.6,0.08,0.6));
#11839=CARTESIAN_POINT('',(-6.60540567951318,0.0874847870182548,-0.3));
#11840=CARTESIAN_POINT('Origin',(-6.665,-0.01,0.6));
#11841=CARTESIAN_POINT('',(-6.65777777777778,0.,-0.3));
#11842=CARTESIAN_POINT('',(-6.65777777777778,0.,0.6));
#11843=CARTESIAN_POINT('',(-6.65777777777778,-1.11022302462516E-16,0.3));
#11844=CARTESIAN_POINT('',(-6.43855476673428,0.303539553752534,-0.3));
#11845=CARTESIAN_POINT('',(-5.5202484787018,1.57504056795133,0.6));
#11846=CARTESIAN_POINT('Origin',(-6.4,0.08,0.6));
#11847=CARTESIAN_POINT('',(-6.34222222222222,0.,0.6));
#11848=CARTESIAN_POINT('',(-6.34222222222222,0.,-0.3));
#11849=CARTESIAN_POINT('',(-6.34222222222222,0.,0.3));
#11850=CARTESIAN_POINT('',(-6.4,0.08,0.6));
#11851=CARTESIAN_POINT('',(-5.28405679513184,-1.46515212981745,0.6));
#11852=CARTESIAN_POINT('',(-6.4,0.08,-0.3));
#11853=CARTESIAN_POINT('',(-6.4,0.08,0.6));
#11854=CARTESIAN_POINT('',(-6.43968559837728,0.134949290060851,-0.3));
#11855=CARTESIAN_POINT('Origin',(-6.465,-0.01,0.6));
#11856=CARTESIAN_POINT('',(-6.45777777777778,0.,-0.3));
#11857=CARTESIAN_POINT('',(-6.45777777777778,0.,0.6));
#11858=CARTESIAN_POINT('',(-6.45777777777778,1.11022302462516E-16,0.3));
#11859=CARTESIAN_POINT('',(-6.27283468559838,0.256075050709939,-0.3));
#11860=CARTESIAN_POINT('',(-5.35452839756591,1.52757606490873,0.6));
#11861=CARTESIAN_POINT('Origin',(-6.,0.08,0.6));
#11862=CARTESIAN_POINT('',(-5.94222222222222,0.,0.6));
#11863=CARTESIAN_POINT('',(-5.94222222222222,0.,-0.3));
#11864=CARTESIAN_POINT('',(-5.94222222222222,2.22044604925031E-16,0.3));
#11865=CARTESIAN_POINT('',(-6.,0.08,0.6));
#11866=CARTESIAN_POINT('',(-4.95261663286005,-1.37022312373225,0.6));
#11867=CARTESIAN_POINT('',(-6.,0.08,-0.3));
#11868=CARTESIAN_POINT('',(-6.,0.08,0.6));
#11869=CARTESIAN_POINT('',(-6.10824543610548,0.229878296146045,-0.3));
#11870=CARTESIAN_POINT('Origin',(-6.065,-0.01,0.6));
#11871=CARTESIAN_POINT('',(-6.05777777777778,0.,-0.3));
#11872=CARTESIAN_POINT('',(-6.05777777777778,0.,0.6));
#11873=CARTESIAN_POINT('',(-6.05777777777778,0.,0.3));
#11874=CARTESIAN_POINT('',(-5.94139452332657,0.161146044624747,-0.3));
#11875=CARTESIAN_POINT('',(-5.02308823529413,1.43264705882353,0.6));
#11876=CARTESIAN_POINT('Origin',(-5.6,0.08,0.6));
#11877=CARTESIAN_POINT('',(-5.54222222222222,0.,0.6));
#11878=CARTESIAN_POINT('',(-5.54222222222222,0.,-0.3));
#11879=CARTESIAN_POINT('',(-5.54222222222222,0.,0.3));
#11880=CARTESIAN_POINT('',(-5.6,0.08,0.6));
#11881=CARTESIAN_POINT('',(-4.62117647058824,-1.27529411764706,0.6));
#11882=CARTESIAN_POINT('',(-5.6,0.08,-0.3));
#11883=CARTESIAN_POINT('',(-5.6,0.08,0.6));
#11884=CARTESIAN_POINT('',(-5.77680527383367,0.324807302231238,-0.3));
#11885=CARTESIAN_POINT('Origin',(-5.665,-0.01,0.6));
#11886=CARTESIAN_POINT('',(-5.65777777777778,0.,-0.3));
#11887=CARTESIAN_POINT('',(-5.65777777777778,0.,0.6));
#11888=CARTESIAN_POINT('',(-5.65777777777778,0.,0.3));
#11889=CARTESIAN_POINT('',(-5.60995436105477,0.066217038539553,-0.3));
#11890=CARTESIAN_POINT('',(-4.6916480730223,1.33771805273834,0.6));
#11891=CARTESIAN_POINT('Origin',(-5.2,0.08,0.6));
#11892=CARTESIAN_POINT('',(-5.14222222222222,0.,0.6));
#11893=CARTESIAN_POINT('',(-5.14222222222222,0.,-0.3));
#11894=CARTESIAN_POINT('',(-5.14222222222222,2.22044604925031E-16,0.3));
#11895=CARTESIAN_POINT('',(-5.2,0.08,0.6));
#11896=CARTESIAN_POINT('',(-4.28973630831642,-1.18036511156187,0.6));
#11897=CARTESIAN_POINT('',(-5.2,0.08,-0.3));
#11898=CARTESIAN_POINT('',(-5.2,0.08,0.6));
#11899=CARTESIAN_POINT('',(-5.44536511156187,0.41973630831643,-0.3));
#11900=CARTESIAN_POINT('Origin',(-5.265,-0.01,0.6));
#11901=CARTESIAN_POINT('',(-5.25777777777778,0.,-0.3));
#11902=CARTESIAN_POINT('',(-5.25777777777778,0.,0.6));
#11903=CARTESIAN_POINT('',(-5.25777777777778,0.,0.3));
#11904=CARTESIAN_POINT('',(-5.27851419878296,-0.0287119675456377,-0.3));
#11905=CARTESIAN_POINT('',(-4.36020791075052,1.24278904665314,0.6));
#11906=CARTESIAN_POINT('Origin',(-4.8,0.08,0.6));
#11907=CARTESIAN_POINT('',(-4.74222222222222,0.,0.6));
#11908=CARTESIAN_POINT('',(-4.74222222222222,0.,-0.3));
#11909=CARTESIAN_POINT('',(-4.74222222222222,2.22044604925031E-16,0.3));
#11910=CARTESIAN_POINT('',(-4.8,0.08,0.6));
#11911=CARTESIAN_POINT('',(-3.95829614604463,-1.08543610547667,0.6));
#11912=CARTESIAN_POINT('',(-4.8,0.08,-0.3));
#11913=CARTESIAN_POINT('',(-4.8,0.08,0.6));
#11914=CARTESIAN_POINT('',(-5.11392494929006,0.514665314401623,-0.3));
#11915=CARTESIAN_POINT('Origin',(-4.865,-0.01,0.6));
#11916=CARTESIAN_POINT('',(-4.85777777777778,0.,-0.3));
#11917=CARTESIAN_POINT('',(-4.85777777777778,0.,0.6));
#11918=CARTESIAN_POINT('',(-4.85777777777778,-2.22044604925031E-16,0.3));
#11919=CARTESIAN_POINT('',(-4.94707403651116,-0.123640973630833,-0.3));
#11920=CARTESIAN_POINT('',(-4.0287677484787,1.14786004056795,0.6));
#11921=CARTESIAN_POINT('Origin',(-4.4,0.08,0.6));
#11922=CARTESIAN_POINT('',(-4.34222222222222,0.,0.6));
#11923=CARTESIAN_POINT('',(-4.34222222222222,0.,-0.3));
#11924=CARTESIAN_POINT('',(-4.34222222222222,0.,0.3));
#11925=CARTESIAN_POINT('',(-4.4,0.08,0.6));
#11926=CARTESIAN_POINT('',(-3.62685598377281,-0.990507099391483,0.6));
#11927=CARTESIAN_POINT('',(-4.4,0.08,-0.3));
#11928=CARTESIAN_POINT('',(-4.4,0.08,0.6));
#11929=CARTESIAN_POINT('',(-4.78248478701826,0.609594320486815,-0.3));
#11930=CARTESIAN_POINT('Origin',(-4.465,-0.01,0.6));
#11931=CARTESIAN_POINT('',(-4.45777777777778,0.,-0.3));
#11932=CARTESIAN_POINT('',(-4.45777777777778,0.,0.6));
#11933=CARTESIAN_POINT('',(-4.45777777777778,0.,0.3));
#11934=CARTESIAN_POINT('',(-4.61563387423935,-0.218569979716023,-0.3));
#11935=CARTESIAN_POINT('',(-3.6973275862069,1.05293103448276,0.6));
#11936=CARTESIAN_POINT('Origin',(-4.,0.08,0.6));
#11937=CARTESIAN_POINT('',(-3.94222222222222,0.,0.6));
#11938=CARTESIAN_POINT('',(-3.94222222222222,0.,-0.3));
#11939=CARTESIAN_POINT('',(-3.94222222222222,0.,0.3));
#11940=CARTESIAN_POINT('',(-4.,0.08,0.6));
#11941=CARTESIAN_POINT('',(-3.29541582150101,-0.895578093306288,0.6));
#11942=CARTESIAN_POINT('',(-4.,0.08,-0.3));
#11943=CARTESIAN_POINT('',(-4.,0.08,0.6));
#11944=CARTESIAN_POINT('',(-4.45104462474645,0.704523326572008,-0.3));
#11945=CARTESIAN_POINT('Origin',(-4.065,-0.01,0.6));
#11946=CARTESIAN_POINT('',(-4.05777777777778,0.,-0.3));
#11947=CARTESIAN_POINT('',(-4.05777777777778,0.,0.6));
#11948=CARTESIAN_POINT('',(-4.05777777777778,-2.22044604925031E-16,0.3));
#11949=CARTESIAN_POINT('',(-4.28419371196754,-0.313498985801215,-0.3));
#11950=CARTESIAN_POINT('',(-3.3658874239351,0.958002028397564,0.6));
#11951=CARTESIAN_POINT('Origin',(-3.6,0.08,0.6));
#11952=CARTESIAN_POINT('',(-3.54222222222222,0.,0.6));
#11953=CARTESIAN_POINT('',(-3.54222222222222,0.,-0.3));
#11954=CARTESIAN_POINT('',(-3.54222222222222,-2.22044604925031E-16,0.3));
#11955=CARTESIAN_POINT('',(-3.6,0.08,0.6));
#11956=CARTESIAN_POINT('',(-2.96397565922921,-0.800649087221095,0.6));
#11957=CARTESIAN_POINT('',(-3.6,0.08,-0.3));
#11958=CARTESIAN_POINT('',(-3.6,0.08,0.6));
#11959=CARTESIAN_POINT('',(-4.11960446247465,0.799452332657201,-0.3));
#11960=CARTESIAN_POINT('Origin',(-3.665,-0.01,0.6));
#11961=CARTESIAN_POINT('',(-3.65777777777778,0.,-0.3));
#11962=CARTESIAN_POINT('',(-3.65777777777778,0.,0.6));
#11963=CARTESIAN_POINT('',(-3.65777777777778,2.22044604925031E-16,0.3));
#11964=CARTESIAN_POINT('',(-3.95275354969574,-0.40842799188641,-0.3));
#11965=CARTESIAN_POINT('',(-3.03444726166329,0.863073022312373,0.6));
#11966=CARTESIAN_POINT('Origin',(-3.2,0.08,0.6));
#11967=CARTESIAN_POINT('',(-3.14222222222222,0.,0.6));
#11968=CARTESIAN_POINT('',(-3.14222222222222,0.,-0.3));
#11969=CARTESIAN_POINT('',(-3.14222222222222,-2.22044604925031E-16,0.3));
#11970=CARTESIAN_POINT('',(-3.2,0.08,0.6));
#11971=CARTESIAN_POINT('',(-2.6325354969574,-0.705720081135902,0.6));
#11972=CARTESIAN_POINT('',(-3.2,0.08,-0.3));
#11973=CARTESIAN_POINT('',(-3.2,0.08,0.6));
#11974=CARTESIAN_POINT('',(-3.78816430020284,0.894381338742393,-0.3));
#11975=CARTESIAN_POINT('Origin',(-3.265,-0.01,0.6));
#11976=CARTESIAN_POINT('',(-3.25777777777778,0.,-0.3));
#11977=CARTESIAN_POINT('',(-3.25777777777778,0.,0.6));
#11978=CARTESIAN_POINT('',(-3.25777777777778,-2.22044604925031E-16,0.3));
#11979=CARTESIAN_POINT('',(-3.62131338742393,-0.5033569979716,-0.3));
#11980=CARTESIAN_POINT('',(-2.70300709939149,0.768144016227179,0.6));
#11981=CARTESIAN_POINT('Origin',(-2.8,0.08,0.6));
#11982=CARTESIAN_POINT('',(-2.74222222222222,0.,0.6));
#11983=CARTESIAN_POINT('',(-2.74222222222222,0.,-0.3));
#11984=CARTESIAN_POINT('',(-2.74222222222222,0.,0.3));
#11985=CARTESIAN_POINT('',(-2.8,0.08,0.6));
#11986=CARTESIAN_POINT('',(-2.3010953346856,-0.610791075050709,0.6));
#11987=CARTESIAN_POINT('',(-2.8,0.08,-0.3));
#11988=CARTESIAN_POINT('',(-2.8,0.08,0.6));
#11989=CARTESIAN_POINT('',(-3.45672413793103,0.989310344827585,-0.3));
#11990=CARTESIAN_POINT('Origin',(-2.865,-0.01,0.6));
#11991=CARTESIAN_POINT('',(-2.85777777777778,0.,-0.3));
#11992=CARTESIAN_POINT('',(-2.85777777777778,0.,0.6));
#11993=CARTESIAN_POINT('',(-2.85777777777778,0.,0.3));
#11994=CARTESIAN_POINT('',(-3.28987322515213,-0.598286004056795,-0.3));
#11995=CARTESIAN_POINT('',(-2.37156693711968,0.673215010141988,0.6));
#11996=CARTESIAN_POINT('Origin',(-10.5,0.,0.));
#11997=CARTESIAN_POINT('',(-1.6,0.,-0.3));
#11998=CARTESIAN_POINT('',(-1.6,0.,-0.3));
#11999=CARTESIAN_POINT('',(-1.6,0.,0.));
#12000=CARTESIAN_POINT('',(-1.6,0.,-0.3));
#12001=CARTESIAN_POINT('',(-1.4,0.,0.));
#12002=CARTESIAN_POINT('',(-1.2,0.,0.));
#12003=CARTESIAN_POINT('',(-1.4,0.,0.6));
#12004=CARTESIAN_POINT('',(-1.4,0.,0.));
#12005=CARTESIAN_POINT('',(-1.2,0.,0.6));
#12006=CARTESIAN_POINT('Origin',(-10.5,0.,0.));
#12007=CARTESIAN_POINT('',(-1.6,0.,-0.3));
#12008=CARTESIAN_POINT('',(-1.2,0.,0.6));
#12009=CARTESIAN_POINT('Origin',(-10.5,0.,0.));
#12010=CARTESIAN_POINT('',(-1.6,0.,-0.3));
#12011=CARTESIAN_POINT('',(-1.2,0.,0.6));
#12012=CARTESIAN_POINT('Origin',(-10.5,0.,0.));
#12013=CARTESIAN_POINT('',(-1.6,0.,-0.3));
#12014=CARTESIAN_POINT('',(-1.2,0.,0.6));
#12015=CARTESIAN_POINT('Origin',(-10.5,0.,0.));
#12016=CARTESIAN_POINT('',(-1.6,0.,-0.3));
#12017=CARTESIAN_POINT('',(-1.2,0.,0.6));
#12018=CARTESIAN_POINT('Origin',(-10.5,0.,0.));
#12019=CARTESIAN_POINT('',(-1.6,0.,-0.3));
#12020=CARTESIAN_POINT('',(-1.2,0.,0.6));
#12021=CARTESIAN_POINT('Origin',(-10.5,0.,0.));
#12022=CARTESIAN_POINT('',(-1.6,0.,-0.3));
#12023=CARTESIAN_POINT('',(-1.2,0.,0.6));
#12024=CARTESIAN_POINT('Origin',(-10.5,0.,0.));
#12025=CARTESIAN_POINT('',(-1.6,0.,-0.3));
#12026=CARTESIAN_POINT('',(-1.2,0.,0.6));
#12027=CARTESIAN_POINT('Origin',(-10.5,0.,0.));
#12028=CARTESIAN_POINT('',(-1.6,0.,-0.3));
#12029=CARTESIAN_POINT('',(-1.2,0.,0.6));
#12030=CARTESIAN_POINT('Origin',(-10.5,0.,0.));
#12031=CARTESIAN_POINT('',(-1.6,0.,-0.3));
#12032=CARTESIAN_POINT('',(-1.2,0.,0.6));
#12033=CARTESIAN_POINT('Origin',(-10.5,0.,0.));
#12034=CARTESIAN_POINT('',(-1.6,0.,-0.3));
#12035=CARTESIAN_POINT('',(-1.2,0.,0.6));
#12036=CARTESIAN_POINT('Origin',(-10.5,0.,0.));
#12037=CARTESIAN_POINT('',(-1.6,0.,-0.3));
#12038=CARTESIAN_POINT('',(-1.2,0.,0.6));
#12039=CARTESIAN_POINT('Origin',(-10.5,0.,0.));
#12040=CARTESIAN_POINT('',(-1.6,0.,-0.3));
#12041=CARTESIAN_POINT('',(-1.2,0.,0.6));
#12042=CARTESIAN_POINT('Origin',(-10.5,0.,0.));
#12043=CARTESIAN_POINT('',(-1.6,0.,-0.3));
#12044=CARTESIAN_POINT('',(-1.2,0.,0.6));
#12045=CARTESIAN_POINT('Origin',(-10.5,0.,0.));
#12046=CARTESIAN_POINT('',(-1.6,0.,-0.3));
#12047=CARTESIAN_POINT('',(-1.2,0.,0.6));
#12048=CARTESIAN_POINT('Origin',(-10.5,0.,0.));
#12049=CARTESIAN_POINT('',(-1.6,0.,-0.3));
#12050=CARTESIAN_POINT('',(-1.2,0.,0.6));
#12051=CARTESIAN_POINT('Origin',(-10.5,0.,0.));
#12052=CARTESIAN_POINT('',(-1.6,0.,-0.3));
#12053=CARTESIAN_POINT('',(-1.2,0.,0.6));
#12054=CARTESIAN_POINT('Origin',(-10.5,0.,0.));
#12055=CARTESIAN_POINT('',(-1.6,0.,-0.3));
#12056=CARTESIAN_POINT('',(-1.2,0.,0.6));
#12057=CARTESIAN_POINT('Origin',(-10.5,0.,0.));
#12058=CARTESIAN_POINT('',(-1.6,0.,-0.3));
#12059=CARTESIAN_POINT('',(-1.2,0.,0.6));
#12060=CARTESIAN_POINT('Origin',(-10.5,0.,0.));
#12061=CARTESIAN_POINT('',(-1.6,0.,-0.3));
#12062=CARTESIAN_POINT('',(-1.2,0.,0.6));
#12063=CARTESIAN_POINT('Origin',(-10.5,0.,0.));
#12064=CARTESIAN_POINT('',(-1.6,0.,-0.3));
#12065=CARTESIAN_POINT('',(-1.2,0.,0.6));
#12066=CARTESIAN_POINT('Origin',(-10.5,0.,0.));
#12067=CARTESIAN_POINT('',(-1.2,0.,0.6));
#12068=CARTESIAN_POINT('',(-1.6,0.,-0.3));
#12069=CARTESIAN_POINT('Origin',(-10.5,0.,0.));
#12070=CARTESIAN_POINT('',(-1.2,0.,0.6));
#12071=CARTESIAN_POINT('',(-1.6,0.,-0.3));
#12072=CARTESIAN_POINT('Origin',(-10.5,0.,0.));
#12073=CARTESIAN_POINT('',(-1.2,0.,0.6));
#12074=CARTESIAN_POINT('',(-1.6,0.,-0.3));
#12075=CARTESIAN_POINT('Origin',(-10.5,0.,0.));
#12076=CARTESIAN_POINT('',(-1.2,0.,0.6));
#12077=CARTESIAN_POINT('',(-1.6,0.,-0.3));
#12078=CARTESIAN_POINT('Origin',(-10.5,0.,0.));
#12079=CARTESIAN_POINT('',(-1.2,0.,0.6));
#12080=CARTESIAN_POINT('',(-1.6,0.,-0.3));
#12081=CARTESIAN_POINT('Origin',(-10.5,0.,0.));
#12082=CARTESIAN_POINT('',(-1.2,0.,0.6));
#12083=CARTESIAN_POINT('',(-1.6,0.,-0.3));
#12084=CARTESIAN_POINT('Origin',(-10.5,0.,0.));
#12085=CARTESIAN_POINT('',(-1.2,0.,0.6));
#12086=CARTESIAN_POINT('',(-1.6,0.,-0.3));
#12087=CARTESIAN_POINT('Origin',(-10.5,0.,0.));
#12088=CARTESIAN_POINT('',(-1.2,0.,0.6));
#12089=CARTESIAN_POINT('',(-1.6,0.,-0.3));
#12090=CARTESIAN_POINT('Origin',(-10.5,0.,0.));
#12091=CARTESIAN_POINT('',(-10.5,0.,0.6));
#12092=CARTESIAN_POINT('',(-1.2,0.,0.6));
#12093=CARTESIAN_POINT('',(-10.5,0.,-0.3));
#12094=CARTESIAN_POINT('',(-10.5,0.,0.));
#12095=CARTESIAN_POINT('',(-1.6,0.,-0.3));
#12096=CARTESIAN_POINT('Origin',(-10.5,0.,0.));
#12097=CARTESIAN_POINT('',(-1.2,0.,0.6));
#12098=CARTESIAN_POINT('',(-1.6,0.,-0.3));
#12099=CARTESIAN_POINT('Origin',(-10.5,0.,0.));
#12100=CARTESIAN_POINT('',(-1.2,0.,0.6));
#12101=CARTESIAN_POINT('',(-1.6,0.,-0.3));
#12102=CARTESIAN_POINT('Origin',(-10.5,0.,0.));
#12103=CARTESIAN_POINT('',(-1.2,0.,0.6));
#12104=CARTESIAN_POINT('',(-1.6,0.,-0.3));
#12105=CARTESIAN_POINT('Origin',(-10.5,0.,0.));
#12106=CARTESIAN_POINT('',(-1.2,0.,0.6));
#12107=CARTESIAN_POINT('',(-1.6,0.,-0.3));
#12108=CARTESIAN_POINT('Origin',(-10.5,0.,0.));
#12109=CARTESIAN_POINT('',(-1.2,0.,0.6));
#12110=CARTESIAN_POINT('',(-1.6,0.,-0.3));
#12111=CARTESIAN_POINT('Origin',(-10.5,0.,0.));
#12112=CARTESIAN_POINT('',(-1.2,0.,0.6));
#12113=CARTESIAN_POINT('',(-1.6,0.,-0.3));
#12114=CARTESIAN_POINT('Origin',(-10.5,0.,0.));
#12115=CARTESIAN_POINT('',(-1.2,0.,0.6));
#12116=CARTESIAN_POINT('',(-1.6,0.,-0.3));
#12117=CARTESIAN_POINT('Origin',(-10.5,0.,0.));
#12118=CARTESIAN_POINT('',(-1.2,0.,0.6));
#12119=CARTESIAN_POINT('',(-1.6,0.,-0.3));
#12120=CARTESIAN_POINT('Origin',(-10.5,0.,0.));
#12121=CARTESIAN_POINT('',(-1.2,0.,0.6));
#12122=CARTESIAN_POINT('',(-1.6,0.,-0.3));
#12123=CARTESIAN_POINT('Origin',(-6.05,0.5,-0.3));
#12124=CARTESIAN_POINT('',(-10.5,0.2,-0.3));
#12125=CARTESIAN_POINT('',(-10.5,0.,-0.3));
#12126=CARTESIAN_POINT('',(-2.8,1.,-0.3));
#12127=CARTESIAN_POINT('',(-10.5,0.2,-0.3));
#12128=CARTESIAN_POINT('',(-1.6,1.,-0.3));
#12129=CARTESIAN_POINT('',(-2.8,1.,-0.3));
#12130=CARTESIAN_POINT('',(-1.6,1.,-0.3));
#12131=CARTESIAN_POINT('Origin',(-1.6,0.,-0.3));
#12132=CARTESIAN_POINT('',(-1.6,1.,0.));
#12133=CARTESIAN_POINT('',(-1.6,1.,-0.3));
#12134=CARTESIAN_POINT('',(-1.6,0.,0.));
#12135=CARTESIAN_POINT('Origin',(-1.2,0.,0.));
#12136=CARTESIAN_POINT('',(-1.2,0.721110255092798,0.));
#12137=CARTESIAN_POINT('',(-1.2,0.721110255092798,0.6));
#12138=CARTESIAN_POINT('',(-1.2,0.721110255092798,0.));
#12139=CARTESIAN_POINT('',(-1.2,1.,0.));
#12140=CARTESIAN_POINT('',(-1.2,1.,0.));
#12141=CARTESIAN_POINT('',(-1.2,1.,0.6));
#12142=CARTESIAN_POINT('',(-1.2,1.,0.));
#12143=CARTESIAN_POINT('',(-1.2,1.,0.6));
#12144=CARTESIAN_POINT('Origin',(-10.5,0.2,0.));
#12145=CARTESIAN_POINT('',(-10.5,0.2,0.6));
#12146=CARTESIAN_POINT('',(-10.5,0.,0.6));
#12147=CARTESIAN_POINT('',(-10.5,0.2,0.));
#12148=CARTESIAN_POINT('Origin',(-2.8,1.,0.));
#12149=CARTESIAN_POINT('',(-2.8,1.,0.6));
#12150=CARTESIAN_POINT('',(-10.5,0.2,0.6));
#12151=CARTESIAN_POINT('',(-2.8,1.,0.));
#12152=CARTESIAN_POINT('Origin',(-1.2,1.,0.));
#12153=CARTESIAN_POINT('',(-2.8,1.,0.6));
#12154=CARTESIAN_POINT('',(-2.8,1.,0.));
#12155=CARTESIAN_POINT('Origin',(0.,0.,0.));
#12156=CARTESIAN_POINT('',(0.993295878967653,0.986591757935306,0.));
#12157=CARTESIAN_POINT('Origin',(0.,0.,0.));
#12158=CARTESIAN_POINT('',(1.,1.,0.));
#12159=CARTESIAN_POINT('',(1.,1.,0.));
#12160=CARTESIAN_POINT('',(3.8,-1.9,0.));
#12161=CARTESIAN_POINT('',(3.8,-1.9,0.));
#12162=CARTESIAN_POINT('',(14.,-1.9,0.));
#12163=CARTESIAN_POINT('',(14.,-1.9,0.));
#12164=CARTESIAN_POINT('',(14.,-3.1,0.));
#12165=CARTESIAN_POINT('',(14.,-3.1,0.));
#12166=CARTESIAN_POINT('',(3.8,-3.1,0.));
#12167=CARTESIAN_POINT('',(3.8,-3.1,0.));
#12168=CARTESIAN_POINT('',(0.533017816115691,-1.29456247732709,0.));
#12169=CARTESIAN_POINT('',(0.,-1.,0.));
#12170=CARTESIAN_POINT('Origin',(0.,0.,0.));
#12171=CARTESIAN_POINT('Origin',(0.,0.,0.));
#12172=CARTESIAN_POINT('',(0.993295878967653,0.986591757935306,0.6));
#12173=CARTESIAN_POINT('Origin',(0.,0.,0.6));
#12174=CARTESIAN_POINT('',(0.993295878967653,0.986591757935306,0.));
#12175=CARTESIAN_POINT('Origin',(0.,-1.,0.));
#12176=CARTESIAN_POINT('',(0.533017816115691,-1.29456247732709,0.6));
#12177=CARTESIAN_POINT('',(0.533017816115691,-1.29456247732709,0.));
#12178=CARTESIAN_POINT('',(3.8,-3.1,0.6));
#12179=CARTESIAN_POINT('',(3.8,-3.1,0.));
#12180=CARTESIAN_POINT('',(0.,-1.,0.6));
#12181=CARTESIAN_POINT('Origin',(1.,1.,0.));
#12182=CARTESIAN_POINT('',(1.,1.,0.6));
#12183=CARTESIAN_POINT('',(1.,1.,0.6));
#12184=CARTESIAN_POINT('',(1.,1.,0.));
#12185=CARTESIAN_POINT('Origin',(3.8,-1.9,0.));
#12186=CARTESIAN_POINT('',(3.8,-1.9,0.6));
#12187=CARTESIAN_POINT('',(3.8,-1.9,0.6));
#12188=CARTESIAN_POINT('',(3.8,-1.9,0.));
#12189=CARTESIAN_POINT('Origin',(14.,-1.9,0.));
#12190=CARTESIAN_POINT('',(14.,-1.9,0.6));
#12191=CARTESIAN_POINT('',(14.,-1.9,0.6));
#12192=CARTESIAN_POINT('',(14.,-1.9,0.));
#12193=CARTESIAN_POINT('Origin',(14.,-3.1,0.));
#12194=CARTESIAN_POINT('',(14.,-3.1,0.6));
#12195=CARTESIAN_POINT('',(14.,-3.1,0.6));
#12196=CARTESIAN_POINT('',(14.,-3.1,0.));
#12197=CARTESIAN_POINT('Origin',(3.8,-3.1,0.));
#12198=CARTESIAN_POINT('',(3.8,-3.1,0.6));
#12199=CARTESIAN_POINT('Origin',(0.,0.,0.6));
#12200=CARTESIAN_POINT('Origin',(0.,0.,0.6));
#12201=CARTESIAN_POINT('Origin',(0.,0.,0.));
#22107=UNCERTAINTY_MEASURE_WITH_UNIT(LENGTH_MEASURE(0.001),#22130,
'DISTANCE_ACCURACY_VALUE',
'Maximum model space distance between geometric entities at asserted c
onnectivities');
#22117=UNCERTAINTY_MEASURE_WITH_UNIT(LENGTH_MEASURE(0.001),#22130,
'DISTANCE_ACCURACY_VALUE',
'Maximum model space distance between geometric entities at asserted c
onnectivities');
#22119=(
GEOMETRIC_REPRESENTATION_CONTEXT(3)
GLOBAL_UNCERTAINTY_ASSIGNED_CONTEXT((#22107))
GLOBAL_UNIT_ASSIGNED_CONTEXT((#22130,#22132,#22133))
REPRESENTATION_CONTEXT('','3D')
);
#22129=(
GEOMETRIC_REPRESENTATION_CONTEXT(3)
GLOBAL_UNCERTAINTY_ASSIGNED_CONTEXT((#22117))
GLOBAL_UNIT_ASSIGNED_CONTEXT((#22130,#22132,#22133))
REPRESENTATION_CONTEXT('','3D')
);
#22130=(
LENGTH_UNIT()
NAMED_UNIT(*)
SI_UNIT(.CENTI.,.METRE.)
);
#22132=(
NAMED_UNIT(*)
PLANE_ANGLE_UNIT()
SI_UNIT($,.RADIAN.)
);
#22133=(
NAMED_UNIT(*)
SI_UNIT($,.STERADIAN.)
SOLID_ANGLE_UNIT()
);
#22135=SHAPE_DEFINITION_REPRESENTATION(#22146,#22173);
#22146=PRODUCT_DEFINITION_SHAPE('',$,#22185);
#22173=SHAPE_REPRESENTATION('',(#8913),#22119);
#22183=PRODUCT_DEFINITION_CONTEXT('part definition',#22218,'design');
#22185=PRODUCT_DEFINITION('Forged jaw and handle',
'Forged jaw and handle',#22196,#22183);
#22196=PRODUCT_DEFINITION_FORMATION('',$,#22221);
#22218=APPLICATION_CONTEXT(
'Core Data for Automotive Mechanical Design Process');
#22219=PRODUCT_CONTEXT('part definition',#22218,'mechanical');
#22221=PRODUCT('Forged jaw and handle','Forged jaw and handle',$,(#22219));
#22232=PRESENTATION_STYLE_ASSIGNMENT((#22240));
#22240=SURFACE_STYLE_USAGE(.BOTH.,#22248);
#22248=SURFACE_SIDE_STYLE('',(#22256));
#22256=SURFACE_STYLE_FILL_AREA(#22264);
#22264=FILL_AREA_STYLE('Tool steel gray',(#22272));
#22272=FILL_AREA_STYLE_COLOUR('Tool steel gray',#22280);
#22280=COLOUR_RGB('Tool steel gray',0.607843137254902,0.643137254901961,
0.698039215686274);
ENDSEC;
END-ISO-10303-21;
